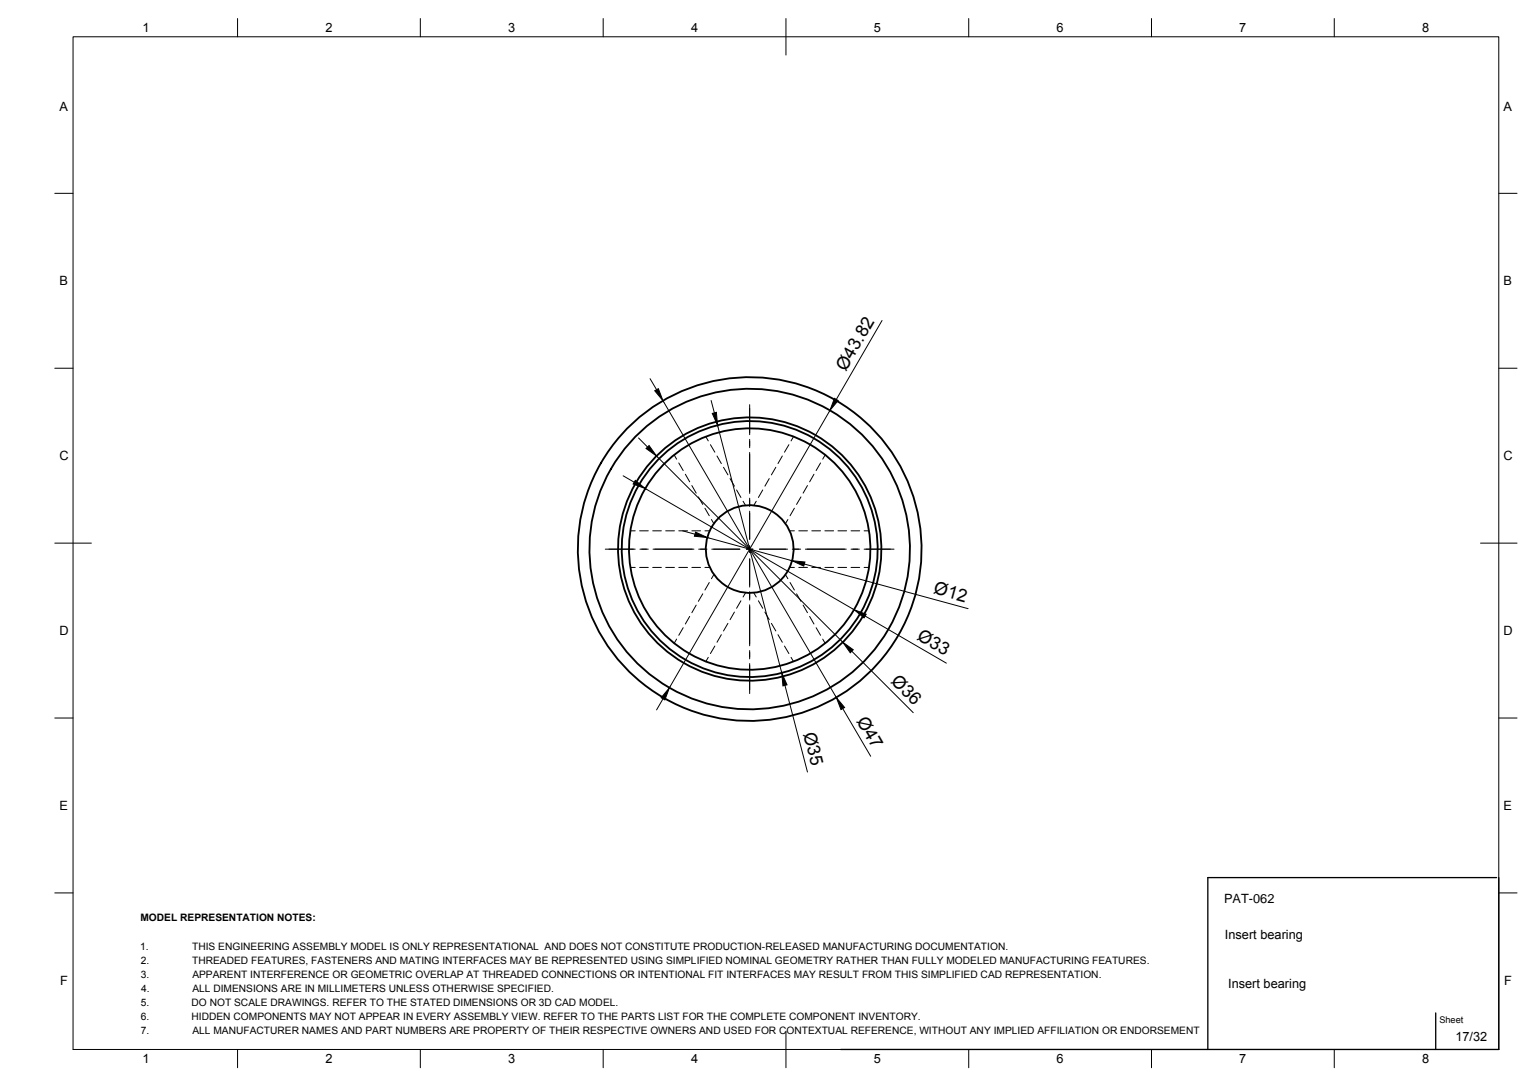
ISO-10303-21;
HEADER;
/* Generated by software containing ST-Developer
 * from STEP Tools, Inc. (www.steptools.com) 
 */

FILE_DESCRIPTION(
/* description */ ('Jaw-coupled motor to shaft test stand'),
/* implementation_level */ '2;1');

FILE_NAME(
/* name */ 'Insert bearing.step',
/* time_stamp */ '2026-10-27T10:46:06-07:00',
/* author */ (''),
/* organization */ (''),
/* preprocessor_version */ 'ST-DEVELOPER v20.2',
/* originating_system */ 'Autodesk Translation Framework v15.17.0.0',
/* authorisation */ '');

FILE_SCHEMA (('AUTOMOTIVE_DESIGN { 1 0 10303 214 3 1 1 }'));
ENDSEC;

DATA;
#10=MECHANICAL_DESIGN_GEOMETRIC_PRESENTATION_REPRESENTATION('',(#354,#355),#19361);
#227=B_SPLINE_CURVE_WITH_KNOTS('',3,(#16151,#16152,#16153,#16154,#16155,
#16156,#16157,#16158,#16159,#16160),.UNSPECIFIED.,.F.,.F.,(4,2,2,2,4),(1.13193471301885,
1.22626174930539,1.32058878559194,1.41491753480854,1.50924628402513),
 .UNSPECIFIED.);
#228=B_SPLINE_CURVE_WITH_KNOTS('',3,(#16162,#16163,#16164,#16165,#16166,
#16167,#16168,#16169,#16170,#16171,#16172,#16173,#16174,#16175,#16176,#16177,
#16178,#16179),.UNSPECIFIED.,.F.,.F.,(4,2,2,2,2,2,2,2,4),(0.377311571006283,
0.471638607292829,0.565965643579376,0.66029439279597,0.754623142012565,
0.84895189122916,0.943280640445754,1.0376076767323,1.13193471301885),
 .UNSPECIFIED.);
#229=B_SPLINE_CURVE_WITH_KNOTS('',3,(#16180,#16181,#16182,#16183,#16184,
#16185,#16186,#16187,#16188,#16189),.UNSPECIFIED.,.F.,.F.,(4,2,2,2,4),(1.50924628402513,
1.60357503324173,1.69790378245832,1.79223081874487,1.88655785503141),
 .UNSPECIFIED.);
#230=B_SPLINE_CURVE_WITH_KNOTS('',3,(#16192,#16193,#16194,#16195,#16196,
#16197,#16198,#16199,#16200,#16201,#16202,#16203,#16204,#16205,#16206,#16207,
#16208,#16209,#16210,#16211,#16212,#16213,#16214,#16215,#16216,#16217,#16218,
#16219,#16220,#16221,#16222,#16223,#16224,#16225),.UNSPECIFIED.,.T.,.F.,
(4,2,2,2,2,2,2,2,2,2,2,2,2,2,2,2,4),(0.,0.0955080856649705,0.191016171329941,
0.286408845249646,0.38180151916935,0.477194193089055,0.572586867008759,
0.66809495267373,0.763603038338701,0.859111124003671,0.954619209668642,
1.05001188358835,1.14540455750805,1.24079723142776,1.33618990534746,1.43169799101243,
1.5272060766774),.UNSPECIFIED.);
#231=B_SPLINE_CURVE_WITH_KNOTS('',3,(#16228,#16229,#16230,#16231,#16232,
#16233,#16234,#16235,#16236,#16237,#16238,#16239,#16240,#16241,#16242,#16243,
#16244,#16245,#16246,#16247,#16248,#16249,#16250,#16251,#16252,#16253,#16254,
#16255,#16256,#16257,#16258,#16259,#16260,#16261),.UNSPECIFIED.,.T.,.F.,
(4,2,2,2,2,2,2,2,2,2,2,2,2,2,2,2,4),(0.,0.0955080856649706,0.191016171329941,
0.286408845249646,0.381801519169351,0.477194193089055,0.57258686700876,
0.668094952673731,0.763603038338701,0.859111124003672,0.954619209668642,
1.05001188358835,1.14540455750805,1.24079723142776,1.33618990534746,1.43169799101243,
1.5272060766774),.UNSPECIFIED.);
#232=B_SPLINE_CURVE_WITH_KNOTS('',3,(#16265,#16266,#16267,#16268,#16269,
#16270,#16271,#16272,#16273,#16274),.UNSPECIFIED.,.F.,.F.,(4,2,2,2,4),(1.13193471301885,
1.22626174930539,1.32058878559194,1.41491753480854,1.50924628402513),
 .UNSPECIFIED.);
#233=B_SPLINE_CURVE_WITH_KNOTS('',3,(#16276,#16277,#16278,#16279,#16280,
#16281,#16282,#16283,#16284,#16285,#16286,#16287,#16288,#16289,#16290,#16291,
#16292,#16293),.UNSPECIFIED.,.F.,.F.,(4,2,2,2,2,2,2,2,4),(0.377311571006283,
0.47163860729283,0.565965643579376,0.660294392795971,0.754623142012565,
0.84895189122916,0.943280640445755,1.0376076767323,1.13193471301885),
 .UNSPECIFIED.);
#234=B_SPLINE_CURVE_WITH_KNOTS('',3,(#16294,#16295,#16296,#16297,#16298,
#16299,#16300,#16301,#16302,#16303),.UNSPECIFIED.,.F.,.F.,(4,2,2,2,4),(1.50924628402513,
1.60357503324173,1.69790378245832,1.79223081874487,1.88655785503141),
 .UNSPECIFIED.);
#235=B_SPLINE_CURVE_WITH_KNOTS('',3,(#16312,#16313,#16314,#16315,#16316,
#16317,#16318,#16319,#16320,#16321,#16322,#16323,#16324,#16325,#16326,#16327,
#16328,#16329),.UNSPECIFIED.,.F.,.F.,(4,2,2,2,2,2,2,2,4),(0.377311571006282,
0.471638607292829,0.565965643579376,0.660294392795971,0.754623142012565,
0.84895189122916,0.943280640445754,1.0376076767323,1.13193471301885),
 .UNSPECIFIED.);
#236=B_SPLINE_CURVE_WITH_KNOTS('',3,(#16331,#16332,#16333,#16334,#16335,
#16336,#16337,#16338,#16339,#16340),.UNSPECIFIED.,.F.,.F.,(4,2,2,2,4),(1.13193471301885,
1.22626174930539,1.32058878559194,1.41491753480854,1.50924628402513),
 .UNSPECIFIED.);
#237=B_SPLINE_CURVE_WITH_KNOTS('',3,(#16341,#16342,#16343,#16344,#16345,
#16346,#16347,#16348,#16349,#16350),.UNSPECIFIED.,.F.,.F.,(4,2,2,2,4),(1.50924628402513,
1.60357503324172,1.69790378245832,1.79223081874487,1.88655785503141),
 .UNSPECIFIED.);
#238=B_SPLINE_CURVE_WITH_KNOTS('',3,(#16353,#16354,#16355,#16356,#16357,
#16358,#16359,#16360,#16361,#16362,#16363,#16364,#16365,#16366,#16367,#16368,
#16369,#16370),.UNSPECIFIED.,.F.,.F.,(4,2,2,2,2,2,2,2,4),(0.377311571006283,
0.47163860729283,0.565965643579376,0.660294392795971,0.754623142012565,
0.84895189122916,0.943280640445754,1.0376076767323,1.13193471301885),
 .UNSPECIFIED.);
#239=B_SPLINE_CURVE_WITH_KNOTS('',3,(#16372,#16373,#16374,#16375,#16376,
#16377,#16378,#16379,#16380,#16381),.UNSPECIFIED.,.F.,.F.,(4,2,2,2,4),(1.13193471301885,
1.22626174930539,1.32058878559194,1.41491753480854,1.50924628402513),
 .UNSPECIFIED.);
#240=B_SPLINE_CURVE_WITH_KNOTS('',3,(#16382,#16383,#16384,#16385,#16386,
#16387,#16388,#16389,#16390,#16391),.UNSPECIFIED.,.F.,.F.,(4,2,2,2,4),(1.50924628402513,
1.60357503324173,1.69790378245832,1.79223081874487,1.88655785503141),
 .UNSPECIFIED.);
#241=B_SPLINE_CURVE_WITH_KNOTS('',3,(#16394,#16395,#16396,#16397,#16398,
#16399,#16400,#16401,#16402,#16403,#16404,#16405,#16406,#16407,#16408,#16409,
#16410,#16411),.UNSPECIFIED.,.F.,.F.,(4,2,2,2,2,2,2,2,4),(0.377311571006282,
0.471638607292829,0.565965643579376,0.66029439279597,0.754623142012565,
0.84895189122916,0.943280640445754,1.0376076767323,1.13193471301885),
 .UNSPECIFIED.);
#242=B_SPLINE_CURVE_WITH_KNOTS('',3,(#16413,#16414,#16415,#16416,#16417,
#16418,#16419,#16420,#16421,#16422),.UNSPECIFIED.,.F.,.F.,(4,2,2,2,4),(1.13193471301885,
1.22626174930539,1.32058878559194,1.41491753480854,1.50924628402513),
 .UNSPECIFIED.);
#243=B_SPLINE_CURVE_WITH_KNOTS('',3,(#16423,#16424,#16425,#16426,#16427,
#16428,#16429,#16430,#16431,#16432),.UNSPECIFIED.,.F.,.F.,(4,2,2,2,4),(1.50924628402513,
1.60357503324172,1.69790378245832,1.79223081874487,1.88655785503141),
 .UNSPECIFIED.);
#244=B_SPLINE_CURVE_WITH_KNOTS('',3,(#16435,#16436,#16437,#16438,#16439,
#16440,#16441,#16442,#16443,#16444,#16445,#16446,#16447,#16448,#16449,#16450,
#16451,#16452),.UNSPECIFIED.,.F.,.F.,(4,2,2,2,2,2,2,2,4),(0.377311571006283,
0.471638607292829,0.565965643579376,0.660294392795971,0.754623142012565,
0.84895189122916,0.943280640445755,1.0376076767323,1.13193471301885),
 .UNSPECIFIED.);
#245=B_SPLINE_CURVE_WITH_KNOTS('',3,(#16454,#16455,#16456,#16457,#16458,
#16459,#16460,#16461,#16462,#16463),.UNSPECIFIED.,.F.,.F.,(4,2,2,2,4),(1.13193471301885,
1.22626174930539,1.32058878559194,1.41491753480854,1.50924628402513),
 .UNSPECIFIED.);
#246=B_SPLINE_CURVE_WITH_KNOTS('',3,(#16464,#16465,#16466,#16467,#16468,
#16469,#16470,#16471,#16472,#16473),.UNSPECIFIED.,.F.,.F.,(4,2,2,2,4),(1.50924628402513,
1.60357503324172,1.69790378245832,1.79223081874487,1.88655785503141),
 .UNSPECIFIED.);
#247=B_SPLINE_CURVE_WITH_KNOTS('',3,(#16477,#16478,#16479,#16480,#16481,
#16482,#16483,#16484,#16485,#16486,#16487,#16488,#16489,#16490,#16491,#16492,
#16493,#16494,#16495,#16496,#16497,#16498,#16499,#16500,#16501,#16502,#16503,
#16504,#16505,#16506,#16507,#16508,#16509,#16510),.UNSPECIFIED.,.T.,.F.,
(4,2,2,2,2,2,2,2,2,2,2,2,2,2,2,2,4),(0.,0.0955080856649705,0.191016171329941,
0.286408845249646,0.38180151916935,0.477194193089055,0.572586867008759,
0.66809495267373,0.7636030383387,0.859111124003671,0.954619209668642,1.05001188358835,
1.14540455750805,1.24079723142776,1.33618990534746,1.43169799101243,1.5272060766774),
 .UNSPECIFIED.);
#248=B_SPLINE_CURVE_WITH_KNOTS('',3,(#16513,#16514,#16515,#16516,#16517,
#16518,#16519,#16520,#16521,#16522,#16523,#16524,#16525,#16526,#16527,#16528,
#16529,#16530,#16531,#16532,#16533,#16534,#16535,#16536,#16537,#16538,#16539,
#16540,#16541,#16542,#16543,#16544,#16545,#16546),.UNSPECIFIED.,.T.,.F.,
(4,2,2,2,2,2,2,2,2,2,2,2,2,2,2,2,4),(0.,0.0955080856649706,0.191016171329941,
0.286408845249646,0.381801519169351,0.477194193089055,0.57258686700876,
0.668094952673731,0.763603038338701,0.859111124003672,0.954619209668642,
1.05001188358835,1.14540455750805,1.24079723142776,1.33618990534746,1.43169799101243,
1.5272060766774),.UNSPECIFIED.);
#249=B_SPLINE_CURVE_WITH_KNOTS('',3,(#16551,#16552,#16553,#16554,#16555,
#16556,#16557,#16558,#16559,#16560,#16561,#16562,#16563,#16564,#16565,#16566,
#16567,#16568,#16569,#16570,#16571,#16572,#16573,#16574,#16575,#16576,#16577,
#16578,#16579,#16580,#16581,#16582,#16583,#16584),.UNSPECIFIED.,.T.,.F.,
(4,2,2,2,2,2,2,2,2,2,2,2,2,2,2,2,4),(0.,0.0955080856649705,0.191016171329941,
0.286408845249646,0.38180151916935,0.477194193089055,0.572586867008759,
0.66809495267373,0.7636030383387,0.859111124003671,0.954619209668642,1.05001188358835,
1.14540455750805,1.24079723142776,1.33618990534746,1.43169799101243,1.5272060766774),
 .UNSPECIFIED.);
#250=B_SPLINE_CURVE_WITH_KNOTS('',3,(#16587,#16588,#16589,#16590,#16591,
#16592,#16593,#16594,#16595,#16596,#16597,#16598,#16599,#16600,#16601,#16602,
#16603,#16604,#16605,#16606,#16607,#16608,#16609,#16610,#16611,#16612,#16613,
#16614,#16615,#16616,#16617,#16618,#16619,#16620),.UNSPECIFIED.,.T.,.F.,
(4,2,2,2,2,2,2,2,2,2,2,2,2,2,2,2,4),(0.,0.0955080856649706,0.191016171329941,
0.286408845249646,0.381801519169351,0.477194193089055,0.57258686700876,
0.668094952673731,0.763603038338701,0.859111124003672,0.954619209668642,
1.05001188358835,1.14540455750805,1.24079723142776,1.33618990534746,1.43169799101243,
1.5272060766774),.UNSPECIFIED.);
#275=SPHERICAL_SURFACE('',#11636,2.35);
#290=SHAPE_REPRESENTATION_RELATIONSHIP('SRR','None',#19505,#322);
#322=ADVANCED_BREP_SHAPE_REPRESENTATION('',(#387,#388),#19341);
#354=STYLED_ITEM('',(#19746),#387);
#355=STYLED_ITEM('',(#19746),#388);
#387=MANIFOLD_SOLID_BREP('Body1',#10998);
#388=MANIFOLD_SOLID_BREP('Body2',#10999);
#460=FACE_BOUND('',#1850,.T.);
#461=FACE_BOUND('',#1852,.T.);
#462=FACE_BOUND('',#1853,.T.);
#463=FACE_BOUND('',#1855,.T.);
#464=FACE_BOUND('',#1859,.T.);
#465=FACE_BOUND('',#1860,.T.);
#466=FACE_BOUND('',#1861,.T.);
#467=FACE_BOUND('',#1862,.T.);
#468=FACE_BOUND('',#1863,.T.);
#469=FACE_BOUND('',#1864,.T.);
#470=FACE_BOUND('',#1870,.T.);
#471=FACE_BOUND('',#1872,.T.);
#472=FACE_BOUND('',#1875,.T.);
#473=FACE_BOUND('',#1877,.T.);
#474=FACE_BOUND('',#1878,.T.);
#475=FACE_BOUND('',#1879,.T.);
#476=FACE_BOUND('',#1880,.T.);
#477=FACE_BOUND('',#1881,.T.);
#478=FACE_BOUND('',#1882,.T.);
#623=PLANE('',#11634);
#624=PLANE('',#11639);
#625=PLANE('',#11649);
#626=PLANE('',#11651);
#627=PLANE('',#11655);
#1171=FACE_OUTER_BOUND('',#1848,.T.);
#1172=FACE_OUTER_BOUND('',#1849,.T.);
#1173=FACE_OUTER_BOUND('',#1851,.T.);
#1174=FACE_OUTER_BOUND('',#1854,.T.);
#1175=FACE_OUTER_BOUND('',#1856,.T.);
#1176=FACE_OUTER_BOUND('',#1857,.T.);
#1177=FACE_OUTER_BOUND('',#1858,.T.);
#1178=FACE_OUTER_BOUND('',#1865,.T.);
#1179=FACE_OUTER_BOUND('',#1866,.T.);
#1180=FACE_OUTER_BOUND('',#1867,.T.);
#1181=FACE_OUTER_BOUND('',#1868,.T.);
#1182=FACE_OUTER_BOUND('',#1869,.T.);
#1183=FACE_OUTER_BOUND('',#1871,.T.);
#1184=FACE_OUTER_BOUND('',#1873,.T.);
#1185=FACE_OUTER_BOUND('',#1874,.T.);
#1186=FACE_OUTER_BOUND('',#1876,.T.);
#1848=EDGE_LOOP('',(#7990,#7991,#7992,#7993));
#1849=EDGE_LOOP('',(#7994));
#1850=EDGE_LOOP('',(#7995));
#1851=EDGE_LOOP('',(#7996,#7997));
#1852=EDGE_LOOP('',(#7998));
#1853=EDGE_LOOP('',(#7999));
#1854=EDGE_LOOP('',(#8000));
#1855=EDGE_LOOP('',(#8001));
#1856=EDGE_LOOP('',(#8002,#8003,#8004,#8005,#8006,#8007));
#1857=EDGE_LOOP('',(#8008,#8009,#8010,#8011,#8012,#8013));
#1858=EDGE_LOOP('',(#8014,#8015,#8016,#8017));
#1859=EDGE_LOOP('',(#8018,#8019,#8020));
#1860=EDGE_LOOP('',(#8021,#8022,#8023));
#1861=EDGE_LOOP('',(#8024,#8025,#8026));
#1862=EDGE_LOOP('',(#8027,#8028,#8029));
#1863=EDGE_LOOP('',(#8030,#8031,#8032));
#1864=EDGE_LOOP('',(#8033,#8034,#8035));
#1865=EDGE_LOOP('',(#8036,#8037,#8038,#8039,#8040,#8041));
#1866=EDGE_LOOP('',(#8042,#8043,#8044,#8045,#8046,#8047));
#1867=EDGE_LOOP('',(#8048,#8049,#8050,#8051,#8052,#8053));
#1868=EDGE_LOOP('',(#8054,#8055,#8056,#8057,#8058,#8059));
#1869=EDGE_LOOP('',(#8060));
#1870=EDGE_LOOP('',(#8061));
#1871=EDGE_LOOP('',(#8062));
#1872=EDGE_LOOP('',(#8063));
#1873=EDGE_LOOP('',(#8064,#8065,#8066,#8067));
#1874=EDGE_LOOP('',(#8068));
#1875=EDGE_LOOP('',(#8069));
#1876=EDGE_LOOP('',(#8070,#8071,#8072,#8073));
#1877=EDGE_LOOP('',(#8074));
#1878=EDGE_LOOP('',(#8075));
#1879=EDGE_LOOP('',(#8076));
#1880=EDGE_LOOP('',(#8077));
#1881=EDGE_LOOP('',(#8078));
#1882=EDGE_LOOP('',(#8079));
#2606=LINE('',#16136,#3759);
#2607=LINE('',#16191,#3760);
#2608=LINE('',#16263,#3761);
#2609=LINE('',#16308,#3762);
#2610=LINE('',#16476,#3763);
#2611=LINE('',#16547,#3764);
#2612=LINE('',#16550,#3765);
#2613=LINE('',#16621,#3766);
#2614=LINE('',#16631,#3767);
#2615=LINE('',#16636,#3768);
#3759=VECTOR('',#13091,1.8);
#3760=VECTOR('',#13108,0.25);
#3761=VECTOR('',#13111,0.25);
#3762=VECTOR('',#13116,1.65);
#3763=VECTOR('',#13121,0.25);
#3764=VECTOR('',#13124,0.25);
#3765=VECTOR('',#13127,0.25);
#3766=VECTOR('',#13130,0.25);
#3767=VECTOR('',#13143,1.75);
#3768=VECTOR('',#13150,0.6);
#4772=CIRCLE('',#11632,1.8);
#4773=CIRCLE('',#11633,1.8);
#4774=CIRCLE('',#11635,2.19089023002066);
#4775=CIRCLE('',#11637,2.35);
#4776=CIRCLE('',#11638,2.19089023002066);
#4777=CIRCLE('',#11643,1.65);
#4778=CIRCLE('',#11644,1.65);
#4779=CIRCLE('',#11650,0.6);
#4780=CIRCLE('',#11652,1.75);
#4781=CIRCLE('',#11654,1.75);
#4782=CIRCLE('',#11656,0.6);
#5159=VERTEX_POINT('',#16133);
#5160=VERTEX_POINT('',#16135);
#5161=VERTEX_POINT('',#16139);
#5162=VERTEX_POINT('',#16142);
#5163=VERTEX_POINT('',#16143);
#5164=VERTEX_POINT('',#16145);
#5165=VERTEX_POINT('',#16149);
#5166=VERTEX_POINT('',#16150);
#5167=VERTEX_POINT('',#16161);
#5168=VERTEX_POINT('',#16190);
#5169=VERTEX_POINT('',#16227);
#5170=VERTEX_POINT('',#16262);
#5171=VERTEX_POINT('',#16264);
#5172=VERTEX_POINT('',#16275);
#5173=VERTEX_POINT('',#16305);
#5174=VERTEX_POINT('',#16307);
#5175=VERTEX_POINT('',#16310);
#5176=VERTEX_POINT('',#16311);
#5177=VERTEX_POINT('',#16330);
#5178=VERTEX_POINT('',#16351);
#5179=VERTEX_POINT('',#16352);
#5180=VERTEX_POINT('',#16371);
#5181=VERTEX_POINT('',#16392);
#5182=VERTEX_POINT('',#16393);
#5183=VERTEX_POINT('',#16412);
#5184=VERTEX_POINT('',#16433);
#5185=VERTEX_POINT('',#16434);
#5186=VERTEX_POINT('',#16453);
#5187=VERTEX_POINT('',#16475);
#5188=VERTEX_POINT('',#16512);
#5189=VERTEX_POINT('',#16549);
#5190=VERTEX_POINT('',#16586);
#5191=VERTEX_POINT('',#16623);
#5192=VERTEX_POINT('',#16626);
#5193=VERTEX_POINT('',#16629);
#5194=VERTEX_POINT('',#16633);
#6206=EDGE_CURVE('',#5159,#5159,#4772,.T.);
#6207=EDGE_CURVE('',#5159,#5160,#2606,.T.);
#6208=EDGE_CURVE('',#5160,#5160,#4773,.T.);
#6209=EDGE_CURVE('',#5161,#5161,#4774,.T.);
#6210=EDGE_CURVE('',#5162,#5163,#4775,.T.);
#6211=EDGE_CURVE('',#5164,#5164,#4776,.T.);
#6212=EDGE_CURVE('',#5165,#5166,#227,.T.);
#6213=EDGE_CURVE('',#5167,#5165,#228,.T.);
#6214=EDGE_CURVE('',#5166,#5167,#229,.T.);
#6215=EDGE_CURVE('',#5166,#5168,#2607,.T.);
#6216=EDGE_CURVE('',#5168,#5168,#230,.T.);
#6217=EDGE_CURVE('',#5169,#5169,#231,.T.);
#6218=EDGE_CURVE('',#5169,#5170,#2608,.T.);
#6219=EDGE_CURVE('',#5171,#5170,#232,.T.);
#6220=EDGE_CURVE('',#5172,#5171,#233,.T.);
#6221=EDGE_CURVE('',#5170,#5172,#234,.T.);
#6222=EDGE_CURVE('',#5173,#5173,#4777,.T.);
#6223=EDGE_CURVE('',#5173,#5174,#2609,.T.);
#6224=EDGE_CURVE('',#5174,#5174,#4778,.T.);
#6225=EDGE_CURVE('',#5175,#5176,#235,.T.);
#6226=EDGE_CURVE('',#5176,#5177,#236,.T.);
#6227=EDGE_CURVE('',#5177,#5175,#237,.T.);
#6228=EDGE_CURVE('',#5178,#5179,#238,.T.);
#6229=EDGE_CURVE('',#5179,#5180,#239,.T.);
#6230=EDGE_CURVE('',#5180,#5178,#240,.T.);
#6231=EDGE_CURVE('',#5181,#5182,#241,.T.);
#6232=EDGE_CURVE('',#5182,#5183,#242,.T.);
#6233=EDGE_CURVE('',#5183,#5181,#243,.T.);
#6234=EDGE_CURVE('',#5184,#5185,#244,.T.);
#6235=EDGE_CURVE('',#5185,#5186,#245,.T.);
#6236=EDGE_CURVE('',#5186,#5184,#246,.T.);
#6237=EDGE_CURVE('',#5177,#5187,#2610,.T.);
#6238=EDGE_CURVE('',#5187,#5187,#247,.T.);
#6239=EDGE_CURVE('',#5188,#5188,#248,.T.);
#6240=EDGE_CURVE('',#5188,#5180,#2611,.T.);
#6241=EDGE_CURVE('',#5183,#5189,#2612,.T.);
#6242=EDGE_CURVE('',#5189,#5189,#249,.T.);
#6243=EDGE_CURVE('',#5190,#5190,#250,.T.);
#6244=EDGE_CURVE('',#5190,#5186,#2613,.T.);
#6245=EDGE_CURVE('',#5191,#5191,#4779,.T.);
#6246=EDGE_CURVE('',#5192,#5192,#4780,.T.);
#6247=EDGE_CURVE('',#5193,#5193,#4781,.T.);
#6248=EDGE_CURVE('',#5193,#5192,#2614,.T.);
#6249=EDGE_CURVE('',#5194,#5194,#4782,.T.);
#6250=EDGE_CURVE('',#5194,#5191,#2615,.T.);
#7990=ORIENTED_EDGE('',*,*,#6206,.T.);
#7991=ORIENTED_EDGE('',*,*,#6207,.T.);
#7992=ORIENTED_EDGE('',*,*,#6208,.F.);
#7993=ORIENTED_EDGE('',*,*,#6207,.F.);
#7994=ORIENTED_EDGE('',*,*,#6209,.F.);
#7995=ORIENTED_EDGE('',*,*,#6208,.T.);
#7996=ORIENTED_EDGE('',*,*,#6210,.T.);
#7997=ORIENTED_EDGE('',*,*,#6210,.F.);
#7998=ORIENTED_EDGE('',*,*,#6209,.T.);
#7999=ORIENTED_EDGE('',*,*,#6211,.F.);
#8000=ORIENTED_EDGE('',*,*,#6211,.T.);
#8001=ORIENTED_EDGE('',*,*,#6206,.F.);
#8002=ORIENTED_EDGE('',*,*,#6212,.F.);
#8003=ORIENTED_EDGE('',*,*,#6213,.F.);
#8004=ORIENTED_EDGE('',*,*,#6214,.F.);
#8005=ORIENTED_EDGE('',*,*,#6215,.T.);
#8006=ORIENTED_EDGE('',*,*,#6216,.F.);
#8007=ORIENTED_EDGE('',*,*,#6215,.F.);
#8008=ORIENTED_EDGE('',*,*,#6217,.F.);
#8009=ORIENTED_EDGE('',*,*,#6218,.T.);
#8010=ORIENTED_EDGE('',*,*,#6219,.F.);
#8011=ORIENTED_EDGE('',*,*,#6220,.F.);
#8012=ORIENTED_EDGE('',*,*,#6221,.F.);
#8013=ORIENTED_EDGE('',*,*,#6218,.F.);
#8014=ORIENTED_EDGE('',*,*,#6222,.F.);
#8015=ORIENTED_EDGE('',*,*,#6223,.T.);
#8016=ORIENTED_EDGE('',*,*,#6224,.T.);
#8017=ORIENTED_EDGE('',*,*,#6223,.F.);
#8018=ORIENTED_EDGE('',*,*,#6213,.T.);
#8019=ORIENTED_EDGE('',*,*,#6212,.T.);
#8020=ORIENTED_EDGE('',*,*,#6214,.T.);
#8021=ORIENTED_EDGE('',*,*,#6220,.T.);
#8022=ORIENTED_EDGE('',*,*,#6219,.T.);
#8023=ORIENTED_EDGE('',*,*,#6221,.T.);
#8024=ORIENTED_EDGE('',*,*,#6225,.T.);
#8025=ORIENTED_EDGE('',*,*,#6226,.T.);
#8026=ORIENTED_EDGE('',*,*,#6227,.T.);
#8027=ORIENTED_EDGE('',*,*,#6228,.T.);
#8028=ORIENTED_EDGE('',*,*,#6229,.T.);
#8029=ORIENTED_EDGE('',*,*,#6230,.T.);
#8030=ORIENTED_EDGE('',*,*,#6231,.T.);
#8031=ORIENTED_EDGE('',*,*,#6232,.T.);
#8032=ORIENTED_EDGE('',*,*,#6233,.T.);
#8033=ORIENTED_EDGE('',*,*,#6234,.T.);
#8034=ORIENTED_EDGE('',*,*,#6235,.T.);
#8035=ORIENTED_EDGE('',*,*,#6236,.T.);
#8036=ORIENTED_EDGE('',*,*,#6226,.F.);
#8037=ORIENTED_EDGE('',*,*,#6225,.F.);
#8038=ORIENTED_EDGE('',*,*,#6227,.F.);
#8039=ORIENTED_EDGE('',*,*,#6237,.T.);
#8040=ORIENTED_EDGE('',*,*,#6238,.F.);
#8041=ORIENTED_EDGE('',*,*,#6237,.F.);
#8042=ORIENTED_EDGE('',*,*,#6239,.F.);
#8043=ORIENTED_EDGE('',*,*,#6240,.T.);
#8044=ORIENTED_EDGE('',*,*,#6229,.F.);
#8045=ORIENTED_EDGE('',*,*,#6228,.F.);
#8046=ORIENTED_EDGE('',*,*,#6230,.F.);
#8047=ORIENTED_EDGE('',*,*,#6240,.F.);
#8048=ORIENTED_EDGE('',*,*,#6232,.F.);
#8049=ORIENTED_EDGE('',*,*,#6231,.F.);
#8050=ORIENTED_EDGE('',*,*,#6233,.F.);
#8051=ORIENTED_EDGE('',*,*,#6241,.T.);
#8052=ORIENTED_EDGE('',*,*,#6242,.F.);
#8053=ORIENTED_EDGE('',*,*,#6241,.F.);
#8054=ORIENTED_EDGE('',*,*,#6243,.F.);
#8055=ORIENTED_EDGE('',*,*,#6244,.T.);
#8056=ORIENTED_EDGE('',*,*,#6235,.F.);
#8057=ORIENTED_EDGE('',*,*,#6234,.F.);
#8058=ORIENTED_EDGE('',*,*,#6236,.F.);
#8059=ORIENTED_EDGE('',*,*,#6244,.F.);
#8060=ORIENTED_EDGE('',*,*,#6224,.F.);
#8061=ORIENTED_EDGE('',*,*,#6245,.T.);
#8062=ORIENTED_EDGE('',*,*,#6246,.F.);
#8063=ORIENTED_EDGE('',*,*,#6222,.T.);
#8064=ORIENTED_EDGE('',*,*,#6247,.F.);
#8065=ORIENTED_EDGE('',*,*,#6248,.T.);
#8066=ORIENTED_EDGE('',*,*,#6246,.T.);
#8067=ORIENTED_EDGE('',*,*,#6248,.F.);
#8068=ORIENTED_EDGE('',*,*,#6247,.T.);
#8069=ORIENTED_EDGE('',*,*,#6249,.F.);
#8070=ORIENTED_EDGE('',*,*,#6249,.T.);
#8071=ORIENTED_EDGE('',*,*,#6250,.T.);
#8072=ORIENTED_EDGE('',*,*,#6245,.F.);
#8073=ORIENTED_EDGE('',*,*,#6250,.F.);
#8074=ORIENTED_EDGE('',*,*,#6217,.T.);
#8075=ORIENTED_EDGE('',*,*,#6216,.T.);
#8076=ORIENTED_EDGE('',*,*,#6239,.T.);
#8077=ORIENTED_EDGE('',*,*,#6238,.T.);
#8078=ORIENTED_EDGE('',*,*,#6243,.T.);
#8079=ORIENTED_EDGE('',*,*,#6242,.T.);
#10311=CYLINDRICAL_SURFACE('',#11631,1.8);
#10312=CYLINDRICAL_SURFACE('',#11640,0.25);
#10313=CYLINDRICAL_SURFACE('',#11641,0.25);
#10314=CYLINDRICAL_SURFACE('',#11642,1.65);
#10315=CYLINDRICAL_SURFACE('',#11645,0.25);
#10316=CYLINDRICAL_SURFACE('',#11646,0.25);
#10317=CYLINDRICAL_SURFACE('',#11647,0.25);
#10318=CYLINDRICAL_SURFACE('',#11648,0.25);
#10319=CYLINDRICAL_SURFACE('',#11653,1.75);
#10320=CYLINDRICAL_SURFACE('',#11657,0.6);
#10513=ADVANCED_FACE('',(#1171),#10311,.F.);
#10514=ADVANCED_FACE('',(#1172,#460),#623,.T.);
#10515=ADVANCED_FACE('',(#1173,#461,#462),#275,.T.);
#10516=ADVANCED_FACE('',(#1174,#463),#624,.T.);
#10517=ADVANCED_FACE('',(#1175),#10312,.F.);
#10518=ADVANCED_FACE('',(#1176),#10313,.F.);
#10519=ADVANCED_FACE('',(#1177,#464,#465,#466,#467,#468,#469),#10314,.T.);
#10520=ADVANCED_FACE('',(#1178),#10315,.F.);
#10521=ADVANCED_FACE('',(#1179),#10316,.F.);
#10522=ADVANCED_FACE('',(#1180),#10317,.F.);
#10523=ADVANCED_FACE('',(#1181),#10318,.F.);
#10524=ADVANCED_FACE('',(#1182,#470),#625,.T.);
#10525=ADVANCED_FACE('',(#1183,#471),#626,.T.);
#10526=ADVANCED_FACE('',(#1184),#10319,.T.);
#10527=ADVANCED_FACE('',(#1185,#472),#627,.T.);
#10528=ADVANCED_FACE('',(#1186,#473,#474,#475,#476,#477,#478),#10320,.F.);
#10998=CLOSED_SHELL('',(#10513,#10514,#10515,#10516));
#10999=CLOSED_SHELL('',(#10517,#10518,#10519,#10520,#10521,#10522,#10523,
#10524,#10525,#10526,#10527,#10528));
#11630=AXIS2_PLACEMENT_3D('',#16131,#13085,#13086);
#11631=AXIS2_PLACEMENT_3D('',#16132,#13087,#13088);
#11632=AXIS2_PLACEMENT_3D('',#16134,#13089,#13090);
#11633=AXIS2_PLACEMENT_3D('',#16137,#13092,#13093);
#11634=AXIS2_PLACEMENT_3D('',#16138,#13094,#13095);
#11635=AXIS2_PLACEMENT_3D('',#16140,#13096,#13097);
#11636=AXIS2_PLACEMENT_3D('',#16141,#13098,#13099);
#11637=AXIS2_PLACEMENT_3D('',#16144,#13100,#13101);
#11638=AXIS2_PLACEMENT_3D('',#16146,#13102,#13103);
#11639=AXIS2_PLACEMENT_3D('',#16147,#13104,#13105);
#11640=AXIS2_PLACEMENT_3D('',#16148,#13106,#13107);
#11641=AXIS2_PLACEMENT_3D('',#16226,#13109,#13110);
#11642=AXIS2_PLACEMENT_3D('',#16304,#13112,#13113);
#11643=AXIS2_PLACEMENT_3D('',#16306,#13114,#13115);
#11644=AXIS2_PLACEMENT_3D('',#16309,#13117,#13118);
#11645=AXIS2_PLACEMENT_3D('',#16474,#13119,#13120);
#11646=AXIS2_PLACEMENT_3D('',#16511,#13122,#13123);
#11647=AXIS2_PLACEMENT_3D('',#16548,#13125,#13126);
#11648=AXIS2_PLACEMENT_3D('',#16585,#13128,#13129);
#11649=AXIS2_PLACEMENT_3D('',#16622,#13131,#13132);
#11650=AXIS2_PLACEMENT_3D('',#16624,#13133,#13134);
#11651=AXIS2_PLACEMENT_3D('',#16625,#13135,#13136);
#11652=AXIS2_PLACEMENT_3D('',#16627,#13137,#13138);
#11653=AXIS2_PLACEMENT_3D('',#16628,#13139,#13140);
#11654=AXIS2_PLACEMENT_3D('',#16630,#13141,#13142);
#11655=AXIS2_PLACEMENT_3D('',#16632,#13144,#13145);
#11656=AXIS2_PLACEMENT_3D('',#16634,#13146,#13147);
#11657=AXIS2_PLACEMENT_3D('',#16635,#13148,#13149);
#13085=DIRECTION('axis',(0.,0.,1.));
#13086=DIRECTION('refdir',(1.,0.,0.));
#13087=DIRECTION('center_axis',(0.,-1.,0.));
#13088=DIRECTION('ref_axis',(1.,0.,0.));
#13089=DIRECTION('center_axis',(0.,-1.,0.));
#13090=DIRECTION('ref_axis',(1.,0.,0.));
#13091=DIRECTION('',(0.,1.,0.));
#13092=DIRECTION('center_axis',(0.,-1.,0.));
#13093=DIRECTION('ref_axis',(1.,0.,0.));
#13094=DIRECTION('center_axis',(0.,1.,0.));
#13095=DIRECTION('ref_axis',(0.,0.,1.));
#13096=DIRECTION('center_axis',(0.,-1.,0.));
#13097=DIRECTION('ref_axis',(1.,0.,0.));
#13098=DIRECTION('center_axis',(6.12323399573677E-17,0.,1.));
#13099=DIRECTION('ref_axis',(1.,0.,0.));
#13100=DIRECTION('center_axis',(1.22464679914735E-16,-1.,0.));
#13101=DIRECTION('ref_axis',(-1.,-1.22464679914735E-16,0.));
#13102=DIRECTION('center_axis',(0.,-1.,0.));
#13103=DIRECTION('ref_axis',(1.,0.,0.));
#13104=DIRECTION('center_axis',(0.,-1.,0.));
#13105=DIRECTION('ref_axis',(0.,0.,-1.));
#13106=DIRECTION('center_axis',(-0.866025403784438,0.,-0.5));
#13107=DIRECTION('ref_axis',(-0.5,0.,0.866025403784438));
#13108=DIRECTION('',(-0.866025403784438,0.,-0.5));
#13109=DIRECTION('center_axis',(-0.866025403784438,0.,-0.5));
#13110=DIRECTION('ref_axis',(-0.5,0.,0.866025403784438));
#13111=DIRECTION('',(-0.866025403784438,0.,-0.5));
#13112=DIRECTION('center_axis',(0.,-1.,0.));
#13113=DIRECTION('ref_axis',(1.,0.,0.));
#13114=DIRECTION('center_axis',(0.,-1.,0.));
#13115=DIRECTION('ref_axis',(1.,0.,0.));
#13116=DIRECTION('',(0.,1.,0.));
#13117=DIRECTION('center_axis',(0.,-1.,0.));
#13118=DIRECTION('ref_axis',(1.,0.,0.));
#13119=DIRECTION('center_axis',(0.866025403784439,0.,-0.5));
#13120=DIRECTION('ref_axis',(-0.5,0.,-0.866025403784439));
#13121=DIRECTION('',(0.866025403784439,0.,-0.5));
#13122=DIRECTION('center_axis',(0.866025403784439,0.,-0.5));
#13123=DIRECTION('ref_axis',(-0.5,0.,-0.866025403784439));
#13124=DIRECTION('',(0.866025403784439,0.,-0.5));
#13125=DIRECTION('center_axis',(0.,0.,1.));
#13126=DIRECTION('ref_axis',(1.,0.,0.));
#13127=DIRECTION('',(0.,0.,1.));
#13128=DIRECTION('center_axis',(0.,0.,1.));
#13129=DIRECTION('ref_axis',(1.,0.,0.));
#13130=DIRECTION('',(0.,0.,1.));
#13131=DIRECTION('center_axis',(0.,1.,0.));
#13132=DIRECTION('ref_axis',(0.,0.,1.));
#13133=DIRECTION('center_axis',(0.,-1.,0.));
#13134=DIRECTION('ref_axis',(1.,0.,0.));
#13135=DIRECTION('center_axis',(0.,1.,0.));
#13136=DIRECTION('ref_axis',(0.,0.,1.));
#13137=DIRECTION('center_axis',(0.,-1.,0.));
#13138=DIRECTION('ref_axis',(1.,0.,0.));
#13139=DIRECTION('center_axis',(0.,-1.,0.));
#13140=DIRECTION('ref_axis',(1.,0.,0.));
#13141=DIRECTION('center_axis',(0.,-1.,0.));
#13142=DIRECTION('ref_axis',(1.,0.,0.));
#13143=DIRECTION('',(0.,1.,0.));
#13144=DIRECTION('center_axis',(0.,-1.,0.));
#13145=DIRECTION('ref_axis',(0.,0.,-1.));
#13146=DIRECTION('center_axis',(0.,-1.,0.));
#13147=DIRECTION('ref_axis',(1.,0.,0.));
#13148=DIRECTION('center_axis',(0.,-1.,0.));
#13149=DIRECTION('ref_axis',(1.,0.,0.));
#13150=DIRECTION('',(0.,1.,0.));
#16131=CARTESIAN_POINT('',(0.,0.,0.));
#16132=CARTESIAN_POINT('Origin',(0.,0.,0.));
#16133=CARTESIAN_POINT('',(-1.8,-0.85,-2.20436423846524E-16));
#16134=CARTESIAN_POINT('Origin',(0.,-0.85,0.));
#16135=CARTESIAN_POINT('',(-1.8,0.85,-2.20436423846524E-16));
#16136=CARTESIAN_POINT('',(-1.8,0.,-2.20436423846524E-16));
#16137=CARTESIAN_POINT('Origin',(0.,0.85,0.));
#16138=CARTESIAN_POINT('Origin',(2.19089023002066,0.85,0.));
#16139=CARTESIAN_POINT('',(2.19089023002066,0.85,0.));
#16140=CARTESIAN_POINT('Origin',(0.,0.85,0.));
#16141=CARTESIAN_POINT('Origin',(3.99680288865056E-15,0.,0.));
#16142=CARTESIAN_POINT('',(3.85290688975075E-15,-1.76221774462768E-32,2.35));
#16143=CARTESIAN_POINT('',(3.85290688975075E-15,-1.76221774462768E-32,-2.35));
#16144=CARTESIAN_POINT('Origin',(3.99680288865056E-15,0.,0.));
#16145=CARTESIAN_POINT('',(2.19089023002066,-0.85,0.));
#16146=CARTESIAN_POINT('Origin',(0.,-0.85,0.));
#16147=CARTESIAN_POINT('Origin',(1.8,-0.85,0.));
#16148=CARTESIAN_POINT('Origin',(0.,1.55,0.));
#16149=CARTESIAN_POINT('',(1.42894191624432,1.8,0.825000000000001));
#16150=CARTESIAN_POINT('',(1.53744468918255,1.55,0.598968970568896));
#16151=CARTESIAN_POINT('Ctrl Pts',(1.42894191624432,1.8,0.825000000000001));
#16152=CARTESIAN_POINT('Ctrl Pts',(1.44466308895875,1.8,0.797770130104052));
#16153=CARTESIAN_POINT('Ctrl Pts',(1.46055812562105,1.79370633789704,0.768258557763732));
#16154=CARTESIAN_POINT('Ctrl Pts',(1.48824888379079,1.76817777258318,0.713138492740816));
#16155=CARTESIAN_POINT('Ctrl Pts',(1.50008999307766,1.74894552961493,0.687551581002689));
#16156=CARTESIAN_POINT('Ctrl Pts',(1.51812136280714,1.70460745840382,0.646764802471699));
#16157=CARTESIAN_POINT('Ctrl Pts',(1.52552758004446,1.67652816181843,0.628833667319578));
#16158=CARTESIAN_POINT('Ctrl Pts',(1.53516661651472,1.61494799959182,0.604921184808251));
#16159=CARTESIAN_POINT('Ctrl Pts',(1.53744468918255,1.58144291640553,0.598968970568896));
#16160=CARTESIAN_POINT('Ctrl Pts',(1.53744468918255,1.55,0.598968970568896));
#16161=CARTESIAN_POINT('',(1.42894191624432,1.3,0.825000000000001));
#16162=CARTESIAN_POINT('Ctrl Pts',(1.42894191624432,1.3,0.825000000000001));
#16163=CARTESIAN_POINT('Ctrl Pts',(1.4132207435299,1.3,0.852229869895949));
#16164=CARTESIAN_POINT('Ctrl Pts',(1.39561049050871,1.30629366210296,0.880751161609749));
#16165=CARTESIAN_POINT('Ctrl Pts',(1.36172049302549,1.33182222741682,0.932292094146256));
#16166=CARTESIAN_POINT('Ctrl Pts',(1.34548213209931,1.35105447038507,0.955340251466734));
#16167=CARTESIAN_POINT('Ctrl Pts',(1.31917543061769,1.39539254159618,0.99134926498299));
#16168=CARTESIAN_POINT('Ctrl Pts',(1.30734972067592,1.42347183818157,1.00672880483252));
#16169=CARTESIAN_POINT('Ctrl Pts',(1.29146042158868,1.48505200040818,1.02703269653942));
#16170=CARTESIAN_POINT('Ctrl Pts',(1.28744468918255,1.51855708359447,1.03198167246111));
#16171=CARTESIAN_POINT('Ctrl Pts',(1.28744468918255,1.58144291640553,1.03198167246111));
#16172=CARTESIAN_POINT('Ctrl Pts',(1.29146042158868,1.61494799959182,1.02703269653942));
#16173=CARTESIAN_POINT('Ctrl Pts',(1.30734972067592,1.67652816181843,1.00672880483252));
#16174=CARTESIAN_POINT('Ctrl Pts',(1.31917543061769,1.70460745840382,0.991349264982991));
#16175=CARTESIAN_POINT('Ctrl Pts',(1.34548213209931,1.74894552961493,0.955340251466735));
#16176=CARTESIAN_POINT('Ctrl Pts',(1.36172049302549,1.76817777258318,0.932292094146256));
#16177=CARTESIAN_POINT('Ctrl Pts',(1.39561049050871,1.79370633789704,0.880751161609749));
#16178=CARTESIAN_POINT('Ctrl Pts',(1.4132207435299,1.8,0.85222986989595));
#16179=CARTESIAN_POINT('Ctrl Pts',(1.42894191624432,1.8,0.825000000000001));
#16180=CARTESIAN_POINT('Ctrl Pts',(1.53744468918255,1.55,0.598968970568896));
#16181=CARTESIAN_POINT('Ctrl Pts',(1.53744468918255,1.51855708359447,0.598968970568896));
#16182=CARTESIAN_POINT('Ctrl Pts',(1.53516661651472,1.48505200040818,0.60492118480825));
#16183=CARTESIAN_POINT('Ctrl Pts',(1.52552758004446,1.42347183818157,0.628833667319578));
#16184=CARTESIAN_POINT('Ctrl Pts',(1.51812136280714,1.39539254159618,0.646764802471699));
#16185=CARTESIAN_POINT('Ctrl Pts',(1.50008999307766,1.35105447038507,0.687551581002689));
#16186=CARTESIAN_POINT('Ctrl Pts',(1.48824888379079,1.33182222741682,0.713138492740816));
#16187=CARTESIAN_POINT('Ctrl Pts',(1.46055812562105,1.30629366210296,0.768258557763732));
#16188=CARTESIAN_POINT('Ctrl Pts',(1.44466308895875,1.3,0.797770130104052));
#16189=CARTESIAN_POINT('Ctrl Pts',(1.42894191624432,1.3,0.825000000000001));
#16190=CARTESIAN_POINT('',(0.59736109069228,1.55,0.0562114519197835));
#16191=CARTESIAN_POINT('',(0.125,1.55,-0.21650635094611));
#16192=CARTESIAN_POINT('Ctrl Pts',(0.59736109069228,1.55,0.0562114519197835));
#16193=CARTESIAN_POINT('Ctrl Pts',(0.59736109069228,1.58183602855499,0.0562114519197835));
#16194=CARTESIAN_POINT('Ctrl Pts',(0.596809586309859,1.61548166177648,0.0633319361811907));
#16195=CARTESIAN_POINT('Ctrl Pts',(0.593243052195919,1.67693412158597,0.0908585874761106));
#16196=CARTESIAN_POINT('Ctrl Pts',(0.590063593315144,1.70478184753241,0.111151766652641));
#16197=CARTESIAN_POINT('Ctrl Pts',(0.579820497891285,1.74874496453875,0.15600214762839));
#16198=CARTESIAN_POINT('Ctrl Pts',(0.572042315803119,1.76792916820474,0.183678633836535));
#16199=CARTESIAN_POINT('Ctrl Pts',(0.549947124580676,1.79356669468566,0.241926459727039));
#16200=CARTESIAN_POINT('Ctrl Pts',(0.53551402125728,1.8,0.27246250701687));
#16201=CARTESIAN_POINT('Ctrl Pts',(0.503716463284046,1.8,0.32753749298313));
#16202=CARTESIAN_POINT('Ctrl Pts',(0.484488022261586,1.79356669468566,0.355304950761552));
#16203=CARTESIAN_POINT('Ctrl Pts',(0.445091520936419,1.76792916820474,0.403563860606914));
#16204=CARTESIAN_POINT('Ctrl Pts',(0.425012071836758,1.74874496453875,0.4241382069946));
#16205=CARTESIAN_POINT('Ctrl Pts',(0.391292050254278,1.70478184753241,0.455434178332924));
#16206=CARTESIAN_POINT('Ctrl Pts',(0.375307371004241,1.67693412158597,0.468334260082228));
#16207=CARTESIAN_POINT('Ctrl Pts',(0.353251858758695,1.61548166177647,0.485186294875824));
#16208=CARTESIAN_POINT('Ctrl Pts',(0.347361090692279,1.58183602855499,0.489224153812003));
#16209=CARTESIAN_POINT('Ctrl Pts',(0.347361090692279,1.51816397144501,0.489224153812003));
#16210=CARTESIAN_POINT('Ctrl Pts',(0.353251858758695,1.48451833822352,0.485186294875824));
#16211=CARTESIAN_POINT('Ctrl Pts',(0.375307371004241,1.42306587841403,0.468334260082228));
#16212=CARTESIAN_POINT('Ctrl Pts',(0.391292050254278,1.39521815246759,0.455434178332924));
#16213=CARTESIAN_POINT('Ctrl Pts',(0.425012071836758,1.35125503546125,0.4241382069946));
#16214=CARTESIAN_POINT('Ctrl Pts',(0.445091520936418,1.33207083179526,0.403563860606914));
#16215=CARTESIAN_POINT('Ctrl Pts',(0.484488022261586,1.30643330531434,0.355304950761552));
#16216=CARTESIAN_POINT('Ctrl Pts',(0.503716463284046,1.3,0.32753749298313));
#16217=CARTESIAN_POINT('Ctrl Pts',(0.53551402125728,1.3,0.27246250701687));
#16218=CARTESIAN_POINT('Ctrl Pts',(0.549947124580676,1.30643330531434,0.241926459727039));
#16219=CARTESIAN_POINT('Ctrl Pts',(0.572042315803119,1.33207083179526,0.183678633836535));
#16220=CARTESIAN_POINT('Ctrl Pts',(0.579820497891285,1.35125503546125,0.15600214762839));
#16221=CARTESIAN_POINT('Ctrl Pts',(0.590063593315144,1.39521815246759,0.111151766652641));
#16222=CARTESIAN_POINT('Ctrl Pts',(0.593243052195919,1.42306587841403,0.0908585874761105));
#16223=CARTESIAN_POINT('Ctrl Pts',(0.596809586309859,1.48451833822352,0.0633319361811906));
#16224=CARTESIAN_POINT('Ctrl Pts',(0.59736109069228,1.51816397144501,0.0562114519197835));
#16225=CARTESIAN_POINT('Ctrl Pts',(0.59736109069228,1.55,0.0562114519197835));
#16226=CARTESIAN_POINT('Origin',(0.,1.55,0.));
#16227=CARTESIAN_POINT('',(-0.347361090692279,1.55,-0.489224153812003));
#16228=CARTESIAN_POINT('Ctrl Pts',(-0.347361090692279,1.55,-0.489224153812003));
#16229=CARTESIAN_POINT('Ctrl Pts',(-0.347361090692279,1.51816397144501,
-0.489224153812003));
#16230=CARTESIAN_POINT('Ctrl Pts',(-0.353251858758695,1.48451833822352,
-0.485186294875824));
#16231=CARTESIAN_POINT('Ctrl Pts',(-0.375307371004241,1.42306587841403,
-0.468334260082228));
#16232=CARTESIAN_POINT('Ctrl Pts',(-0.391292050254278,1.39521815246759,
-0.455434178332924));
#16233=CARTESIAN_POINT('Ctrl Pts',(-0.425012071836758,1.35125503546125,
-0.4241382069946));
#16234=CARTESIAN_POINT('Ctrl Pts',(-0.445091520936419,1.33207083179526,
-0.403563860606914));
#16235=CARTESIAN_POINT('Ctrl Pts',(-0.484488022261586,1.30643330531434,
-0.355304950761552));
#16236=CARTESIAN_POINT('Ctrl Pts',(-0.503716463284046,1.3,-0.32753749298313));
#16237=CARTESIAN_POINT('Ctrl Pts',(-0.53551402125728,1.3,-0.27246250701687));
#16238=CARTESIAN_POINT('Ctrl Pts',(-0.549947124580676,1.30643330531434,
-0.241926459727039));
#16239=CARTESIAN_POINT('Ctrl Pts',(-0.572042315803119,1.33207083179526,
-0.183678633836535));
#16240=CARTESIAN_POINT('Ctrl Pts',(-0.579820497891285,1.35125503546125,
-0.15600214762839));
#16241=CARTESIAN_POINT('Ctrl Pts',(-0.590063593315144,1.39521815246759,
-0.111151766652641));
#16242=CARTESIAN_POINT('Ctrl Pts',(-0.593243052195918,1.42306587841403,
-0.0908585874761106));
#16243=CARTESIAN_POINT('Ctrl Pts',(-0.596809586309859,1.48451833822352,
-0.0633319361811906));
#16244=CARTESIAN_POINT('Ctrl Pts',(-0.597361090692279,1.51816397144501,
-0.0562114519197835));
#16245=CARTESIAN_POINT('Ctrl Pts',(-0.597361090692279,1.58183602855499,
-0.0562114519197835));
#16246=CARTESIAN_POINT('Ctrl Pts',(-0.596809586309859,1.61548166177647,
-0.0633319361811905));
#16247=CARTESIAN_POINT('Ctrl Pts',(-0.593243052195918,1.67693412158597,
-0.0908585874761104));
#16248=CARTESIAN_POINT('Ctrl Pts',(-0.590063593315144,1.70478184753241,
-0.111151766652641));
#16249=CARTESIAN_POINT('Ctrl Pts',(-0.579820497891285,1.74874496453875,
-0.15600214762839));
#16250=CARTESIAN_POINT('Ctrl Pts',(-0.572042315803118,1.76792916820474,
-0.183678633836535));
#16251=CARTESIAN_POINT('Ctrl Pts',(-0.549947124580676,1.79356669468566,
-0.241926459727039));
#16252=CARTESIAN_POINT('Ctrl Pts',(-0.53551402125728,1.8,-0.27246250701687));
#16253=CARTESIAN_POINT('Ctrl Pts',(-0.503716463284046,1.8,-0.32753749298313));
#16254=CARTESIAN_POINT('Ctrl Pts',(-0.484488022261586,1.79356669468566,
-0.355304950761552));
#16255=CARTESIAN_POINT('Ctrl Pts',(-0.445091520936419,1.76792916820474,
-0.403563860606914));
#16256=CARTESIAN_POINT('Ctrl Pts',(-0.425012071836758,1.74874496453875,
-0.4241382069946));
#16257=CARTESIAN_POINT('Ctrl Pts',(-0.391292050254278,1.70478184753241,
-0.455434178332924));
#16258=CARTESIAN_POINT('Ctrl Pts',(-0.375307371004241,1.67693412158597,
-0.468334260082228));
#16259=CARTESIAN_POINT('Ctrl Pts',(-0.353251858758695,1.61548166177648,
-0.485186294875824));
#16260=CARTESIAN_POINT('Ctrl Pts',(-0.347361090692279,1.58183602855499,
-0.489224153812003));
#16261=CARTESIAN_POINT('Ctrl Pts',(-0.347361090692279,1.55,-0.489224153812003));
#16262=CARTESIAN_POINT('',(-1.28744468918255,1.55,-1.03198167246111));
#16263=CARTESIAN_POINT('',(0.125,1.55,-0.21650635094611));
#16264=CARTESIAN_POINT('',(-1.42894191624432,1.3,-0.825000000000001));
#16265=CARTESIAN_POINT('Ctrl Pts',(-1.42894191624432,1.3,-0.825000000000001));
#16266=CARTESIAN_POINT('Ctrl Pts',(-1.4132207435299,1.3,-0.852229869895949));
#16267=CARTESIAN_POINT('Ctrl Pts',(-1.39561049050871,1.30629366210296,-0.880751161609749));
#16268=CARTESIAN_POINT('Ctrl Pts',(-1.36172049302549,1.33182222741682,-0.932292094146256));
#16269=CARTESIAN_POINT('Ctrl Pts',(-1.34548213209931,1.35105447038507,-0.955340251466735));
#16270=CARTESIAN_POINT('Ctrl Pts',(-1.31917543061769,1.39539254159618,-0.991349264982991));
#16271=CARTESIAN_POINT('Ctrl Pts',(-1.30734972067592,1.42347183818157,-1.00672880483252));
#16272=CARTESIAN_POINT('Ctrl Pts',(-1.29146042158868,1.48505200040818,-1.02703269653942));
#16273=CARTESIAN_POINT('Ctrl Pts',(-1.28744468918255,1.51855708359447,-1.03198167246111));
#16274=CARTESIAN_POINT('Ctrl Pts',(-1.28744468918255,1.55,-1.03198167246111));
#16275=CARTESIAN_POINT('',(-1.42894191624432,1.8,-0.825000000000001));
#16276=CARTESIAN_POINT('Ctrl Pts',(-1.42894191624432,1.8,-0.825000000000001));
#16277=CARTESIAN_POINT('Ctrl Pts',(-1.44466308895875,1.8,-0.797770130104052));
#16278=CARTESIAN_POINT('Ctrl Pts',(-1.46055812562105,1.79370633789704,-0.768258557763732));
#16279=CARTESIAN_POINT('Ctrl Pts',(-1.48824888379079,1.76817777258318,-0.713138492740816));
#16280=CARTESIAN_POINT('Ctrl Pts',(-1.50008999307766,1.74894552961493,-0.687551581002689));
#16281=CARTESIAN_POINT('Ctrl Pts',(-1.51812136280714,1.70460745840382,-0.646764802471699));
#16282=CARTESIAN_POINT('Ctrl Pts',(-1.52552758004446,1.67652816181843,-0.628833667319578));
#16283=CARTESIAN_POINT('Ctrl Pts',(-1.53516661651472,1.61494799959182,-0.60492118480825));
#16284=CARTESIAN_POINT('Ctrl Pts',(-1.53744468918255,1.58144291640553,-0.598968970568896));
#16285=CARTESIAN_POINT('Ctrl Pts',(-1.53744468918255,1.51855708359447,-0.598968970568896));
#16286=CARTESIAN_POINT('Ctrl Pts',(-1.53516661651472,1.48505200040818,-0.60492118480825));
#16287=CARTESIAN_POINT('Ctrl Pts',(-1.52552758004446,1.42347183818157,-0.628833667319578));
#16288=CARTESIAN_POINT('Ctrl Pts',(-1.51812136280714,1.39539254159618,-0.646764802471699));
#16289=CARTESIAN_POINT('Ctrl Pts',(-1.50008999307766,1.35105447038507,-0.687551581002689));
#16290=CARTESIAN_POINT('Ctrl Pts',(-1.48824888379079,1.33182222741682,-0.713138492740816));
#16291=CARTESIAN_POINT('Ctrl Pts',(-1.46055812562105,1.30629366210296,-0.768258557763732));
#16292=CARTESIAN_POINT('Ctrl Pts',(-1.44466308895875,1.3,-0.797770130104052));
#16293=CARTESIAN_POINT('Ctrl Pts',(-1.42894191624432,1.3,-0.825000000000001));
#16294=CARTESIAN_POINT('Ctrl Pts',(-1.28744468918255,1.55,-1.03198167246111));
#16295=CARTESIAN_POINT('Ctrl Pts',(-1.28744468918255,1.58144291640553,-1.03198167246111));
#16296=CARTESIAN_POINT('Ctrl Pts',(-1.29146042158868,1.61494799959182,-1.02703269653942));
#16297=CARTESIAN_POINT('Ctrl Pts',(-1.30734972067592,1.67652816181843,-1.00672880483252));
#16298=CARTESIAN_POINT('Ctrl Pts',(-1.31917543061769,1.70460745840382,-0.991349264982991));
#16299=CARTESIAN_POINT('Ctrl Pts',(-1.34548213209931,1.74894552961493,-0.955340251466734));
#16300=CARTESIAN_POINT('Ctrl Pts',(-1.36172049302549,1.76817777258318,-0.932292094146256));
#16301=CARTESIAN_POINT('Ctrl Pts',(-1.39561049050871,1.79370633789704,-0.880751161609749));
#16302=CARTESIAN_POINT('Ctrl Pts',(-1.4132207435299,1.8,-0.852229869895949));
#16303=CARTESIAN_POINT('Ctrl Pts',(-1.42894191624432,1.8,-0.825000000000001));
#16304=CARTESIAN_POINT('Origin',(0.,1.55,0.));
#16305=CARTESIAN_POINT('',(-1.65,0.85,-2.02066721859313E-16));
#16306=CARTESIAN_POINT('Origin',(0.,0.85,0.));
#16307=CARTESIAN_POINT('',(-1.65,2.25,-2.02066721859313E-16));
#16308=CARTESIAN_POINT('',(-1.65,1.55,-2.02066721859313E-16));
#16309=CARTESIAN_POINT('Origin',(0.,2.25,0.));
#16310=CARTESIAN_POINT('',(-1.42894191624432,1.3,0.825));
#16311=CARTESIAN_POINT('',(-1.42894191624432,1.8,0.825));
#16312=CARTESIAN_POINT('Ctrl Pts',(-1.42894191624432,1.3,0.825));
#16313=CARTESIAN_POINT('Ctrl Pts',(-1.44466308895875,1.3,0.797770130104051));
#16314=CARTESIAN_POINT('Ctrl Pts',(-1.46055812562105,1.30629366210296,0.768258557763731));
#16315=CARTESIAN_POINT('Ctrl Pts',(-1.48824888379079,1.33182222741682,0.713138492740815));
#16316=CARTESIAN_POINT('Ctrl Pts',(-1.50008999307766,1.35105447038507,0.687551581002688));
#16317=CARTESIAN_POINT('Ctrl Pts',(-1.51812136280714,1.39539254159618,0.646764802471698));
#16318=CARTESIAN_POINT('Ctrl Pts',(-1.52552758004446,1.42347183818157,0.628833667319577));
#16319=CARTESIAN_POINT('Ctrl Pts',(-1.53516661651472,1.48505200040818,0.604921184808249));
#16320=CARTESIAN_POINT('Ctrl Pts',(-1.53744468918255,1.51855708359447,0.598968970568895));
#16321=CARTESIAN_POINT('Ctrl Pts',(-1.53744468918255,1.58144291640553,0.598968970568895));
#16322=CARTESIAN_POINT('Ctrl Pts',(-1.53516661651472,1.61494799959182,0.604921184808249));
#16323=CARTESIAN_POINT('Ctrl Pts',(-1.52552758004446,1.67652816181843,0.628833667319577));
#16324=CARTESIAN_POINT('Ctrl Pts',(-1.51812136280714,1.70460745840382,0.646764802471698));
#16325=CARTESIAN_POINT('Ctrl Pts',(-1.50008999307766,1.74894552961493,0.687551581002688));
#16326=CARTESIAN_POINT('Ctrl Pts',(-1.48824888379079,1.76817777258318,0.713138492740815));
#16327=CARTESIAN_POINT('Ctrl Pts',(-1.46055812562105,1.79370633789704,0.768258557763731));
#16328=CARTESIAN_POINT('Ctrl Pts',(-1.44466308895875,1.8,0.797770130104051));
#16329=CARTESIAN_POINT('Ctrl Pts',(-1.42894191624432,1.8,0.825));
#16330=CARTESIAN_POINT('',(-1.28744468918255,1.55,1.03198167246111));
#16331=CARTESIAN_POINT('Ctrl Pts',(-1.42894191624432,1.8,0.825));
#16332=CARTESIAN_POINT('Ctrl Pts',(-1.4132207435299,1.8,0.852229869895948));
#16333=CARTESIAN_POINT('Ctrl Pts',(-1.39561049050871,1.79370633789704,0.880751161609747));
#16334=CARTESIAN_POINT('Ctrl Pts',(-1.36172049302549,1.76817777258318,0.932292094146255));
#16335=CARTESIAN_POINT('Ctrl Pts',(-1.34548213209931,1.74894552961493,0.955340251466733));
#16336=CARTESIAN_POINT('Ctrl Pts',(-1.31917543061769,1.70460745840382,0.991349264982989));
#16337=CARTESIAN_POINT('Ctrl Pts',(-1.30734972067592,1.67652816181843,1.00672880483252));
#16338=CARTESIAN_POINT('Ctrl Pts',(-1.29146042158868,1.61494799959182,1.02703269653942));
#16339=CARTESIAN_POINT('Ctrl Pts',(-1.28744468918255,1.58144291640553,1.03198167246111));
#16340=CARTESIAN_POINT('Ctrl Pts',(-1.28744468918255,1.55,1.03198167246111));
#16341=CARTESIAN_POINT('Ctrl Pts',(-1.28744468918255,1.55,1.03198167246111));
#16342=CARTESIAN_POINT('Ctrl Pts',(-1.28744468918255,1.51855708359447,1.03198167246111));
#16343=CARTESIAN_POINT('Ctrl Pts',(-1.29146042158868,1.48505200040818,1.02703269653942));
#16344=CARTESIAN_POINT('Ctrl Pts',(-1.30734972067592,1.42347183818157,1.00672880483252));
#16345=CARTESIAN_POINT('Ctrl Pts',(-1.31917543061769,1.39539254159618,0.99134926498299));
#16346=CARTESIAN_POINT('Ctrl Pts',(-1.34548213209931,1.35105447038508,0.955340251466733));
#16347=CARTESIAN_POINT('Ctrl Pts',(-1.36172049302549,1.33182222741682,0.932292094146255));
#16348=CARTESIAN_POINT('Ctrl Pts',(-1.39561049050871,1.30629366210296,0.880751161609748));
#16349=CARTESIAN_POINT('Ctrl Pts',(-1.4132207435299,1.3,0.852229869895949));
#16350=CARTESIAN_POINT('Ctrl Pts',(-1.42894191624432,1.3,0.825));
#16351=CARTESIAN_POINT('',(1.42894191624432,1.8,-0.825));
#16352=CARTESIAN_POINT('',(1.42894191624432,1.3,-0.825));
#16353=CARTESIAN_POINT('Ctrl Pts',(1.42894191624432,1.8,-0.825));
#16354=CARTESIAN_POINT('Ctrl Pts',(1.4132207435299,1.8,-0.852229869895949));
#16355=CARTESIAN_POINT('Ctrl Pts',(1.39561049050871,1.79370633789704,-0.880751161609748));
#16356=CARTESIAN_POINT('Ctrl Pts',(1.36172049302549,1.76817777258318,-0.932292094146255));
#16357=CARTESIAN_POINT('Ctrl Pts',(1.34548213209931,1.74894552961493,-0.955340251466734));
#16358=CARTESIAN_POINT('Ctrl Pts',(1.31917543061769,1.70460745840382,-0.99134926498299));
#16359=CARTESIAN_POINT('Ctrl Pts',(1.30734972067592,1.67652816181843,-1.00672880483252));
#16360=CARTESIAN_POINT('Ctrl Pts',(1.29146042158868,1.61494799959182,-1.02703269653942));
#16361=CARTESIAN_POINT('Ctrl Pts',(1.28744468918255,1.58144291640553,-1.03198167246111));
#16362=CARTESIAN_POINT('Ctrl Pts',(1.28744468918255,1.51855708359447,-1.03198167246111));
#16363=CARTESIAN_POINT('Ctrl Pts',(1.29146042158868,1.48505200040818,-1.02703269653942));
#16364=CARTESIAN_POINT('Ctrl Pts',(1.30734972067592,1.42347183818157,-1.00672880483252));
#16365=CARTESIAN_POINT('Ctrl Pts',(1.31917543061769,1.39539254159618,-0.99134926498299));
#16366=CARTESIAN_POINT('Ctrl Pts',(1.34548213209931,1.35105447038507,-0.955340251466734));
#16367=CARTESIAN_POINT('Ctrl Pts',(1.36172049302549,1.33182222741682,-0.932292094146255));
#16368=CARTESIAN_POINT('Ctrl Pts',(1.39561049050871,1.30629366210296,-0.880751161609748));
#16369=CARTESIAN_POINT('Ctrl Pts',(1.4132207435299,1.3,-0.852229869895948));
#16370=CARTESIAN_POINT('Ctrl Pts',(1.42894191624432,1.3,-0.825));
#16371=CARTESIAN_POINT('',(1.53744468918255,1.55,-0.598968970568895));
#16372=CARTESIAN_POINT('Ctrl Pts',(1.42894191624432,1.3,-0.825));
#16373=CARTESIAN_POINT('Ctrl Pts',(1.44466308895875,1.3,-0.797770130104051));
#16374=CARTESIAN_POINT('Ctrl Pts',(1.46055812562105,1.30629366210296,-0.768258557763731));
#16375=CARTESIAN_POINT('Ctrl Pts',(1.48824888379079,1.33182222741682,-0.713138492740815));
#16376=CARTESIAN_POINT('Ctrl Pts',(1.50008999307766,1.35105447038507,-0.687551581002688));
#16377=CARTESIAN_POINT('Ctrl Pts',(1.51812136280714,1.39539254159618,-0.646764802471698));
#16378=CARTESIAN_POINT('Ctrl Pts',(1.52552758004446,1.42347183818157,-0.628833667319577));
#16379=CARTESIAN_POINT('Ctrl Pts',(1.53516661651472,1.48505200040818,-0.604921184808249));
#16380=CARTESIAN_POINT('Ctrl Pts',(1.53744468918255,1.51855708359447,-0.598968970568895));
#16381=CARTESIAN_POINT('Ctrl Pts',(1.53744468918255,1.55,-0.598968970568895));
#16382=CARTESIAN_POINT('Ctrl Pts',(1.53744468918255,1.55,-0.598968970568895));
#16383=CARTESIAN_POINT('Ctrl Pts',(1.53744468918255,1.58144291640553,-0.598968970568895));
#16384=CARTESIAN_POINT('Ctrl Pts',(1.53516661651472,1.61494799959182,-0.604921184808249));
#16385=CARTESIAN_POINT('Ctrl Pts',(1.52552758004446,1.67652816181843,-0.628833667319577));
#16386=CARTESIAN_POINT('Ctrl Pts',(1.51812136280714,1.70460745840382,-0.646764802471698));
#16387=CARTESIAN_POINT('Ctrl Pts',(1.50008999307766,1.74894552961493,-0.687551581002688));
#16388=CARTESIAN_POINT('Ctrl Pts',(1.48824888379079,1.76817777258318,-0.713138492740815));
#16389=CARTESIAN_POINT('Ctrl Pts',(1.46055812562105,1.79370633789704,-0.768258557763731));
#16390=CARTESIAN_POINT('Ctrl Pts',(1.44466308895875,1.8,-0.797770130104051));
#16391=CARTESIAN_POINT('Ctrl Pts',(1.42894191624432,1.8,-0.825));
#16392=CARTESIAN_POINT('',(0.,1.3,-1.65));
#16393=CARTESIAN_POINT('',(0.,1.8,-1.65));
#16394=CARTESIAN_POINT('Ctrl Pts',(1.38777878078145E-17,1.3,-1.65));
#16395=CARTESIAN_POINT('Ctrl Pts',(0.0314423454288489,1.3,-1.65));
#16396=CARTESIAN_POINT('Ctrl Pts',(0.0649476351123396,1.30629366210296,
-1.64900971937348));
#16397=CARTESIAN_POINT('Ctrl Pts',(0.126528390765307,1.33182222741682,-1.64543058688707));
#16398=CARTESIAN_POINT('Ctrl Pts',(0.154607860978348,1.35105447038507,-1.64289183246942));
#16399=CARTESIAN_POINT('Ctrl Pts',(0.198945932189457,1.39539254159618,-1.63811406745469));
#16400=CARTESIAN_POINT('Ctrl Pts',(0.218177859368546,1.42347183818157,-1.63556247215209));
#16401=CARTESIAN_POINT('Ctrl Pts',(0.243706194926033,1.48505200040818,-1.63195388134767));
#16402=CARTESIAN_POINT('Ctrl Pts',(0.25,1.51855708359447,-1.63095064303001));
#16403=CARTESIAN_POINT('Ctrl Pts',(0.25,1.58144291640553,-1.63095064303001));
#16404=CARTESIAN_POINT('Ctrl Pts',(0.243706194926033,1.61494799959182,-1.63195388134767));
#16405=CARTESIAN_POINT('Ctrl Pts',(0.218177859368546,1.67652816181843,-1.63556247215209));
#16406=CARTESIAN_POINT('Ctrl Pts',(0.198945932189457,1.70460745840382,-1.63811406745469));
#16407=CARTESIAN_POINT('Ctrl Pts',(0.154607860978349,1.74894552961493,-1.64289183246942));
#16408=CARTESIAN_POINT('Ctrl Pts',(0.126528390765307,1.76817777258318,-1.64543058688707));
#16409=CARTESIAN_POINT('Ctrl Pts',(0.0649476351123398,1.79370633789704,
-1.64900971937348));
#16410=CARTESIAN_POINT('Ctrl Pts',(0.031442345428849,1.8,-1.65));
#16411=CARTESIAN_POINT('Ctrl Pts',(7.63278329429795E-17,1.8,-1.65));
#16412=CARTESIAN_POINT('',(-0.25,1.55,-1.63095064303001));
#16413=CARTESIAN_POINT('Ctrl Pts',(9.0205620750794E-17,1.8,-1.65));
#16414=CARTESIAN_POINT('Ctrl Pts',(-0.0314423454288488,1.8,-1.65));
#16415=CARTESIAN_POINT('Ctrl Pts',(-0.0649476351123396,1.79370633789704,
-1.64900971937348));
#16416=CARTESIAN_POINT('Ctrl Pts',(-0.126528390765307,1.76817777258318,
-1.64543058688707));
#16417=CARTESIAN_POINT('Ctrl Pts',(-0.154607860978348,1.74894552961493,
-1.64289183246942));
#16418=CARTESIAN_POINT('Ctrl Pts',(-0.198945932189456,1.70460745840382,
-1.63811406745469));
#16419=CARTESIAN_POINT('Ctrl Pts',(-0.218177859368546,1.67652816181843,
-1.63556247215209));
#16420=CARTESIAN_POINT('Ctrl Pts',(-0.243706194926033,1.61494799959182,
-1.63195388134767));
#16421=CARTESIAN_POINT('Ctrl Pts',(-0.25,1.58144291640553,-1.63095064303001));
#16422=CARTESIAN_POINT('Ctrl Pts',(-0.25,1.55,-1.63095064303001));
#16423=CARTESIAN_POINT('Ctrl Pts',(-0.25,1.55,-1.63095064303001));
#16424=CARTESIAN_POINT('Ctrl Pts',(-0.25,1.51855708359447,-1.63095064303001));
#16425=CARTESIAN_POINT('Ctrl Pts',(-0.243706194926033,1.48505200040818,
-1.63195388134767));
#16426=CARTESIAN_POINT('Ctrl Pts',(-0.218177859368546,1.42347183818157,
-1.63556247215209));
#16427=CARTESIAN_POINT('Ctrl Pts',(-0.198945932189457,1.39539254159618,
-1.63811406745469));
#16428=CARTESIAN_POINT('Ctrl Pts',(-0.154607860978349,1.35105447038507,
-1.64289183246942));
#16429=CARTESIAN_POINT('Ctrl Pts',(-0.126528390765307,1.33182222741682,
-1.64543058688707));
#16430=CARTESIAN_POINT('Ctrl Pts',(-0.0649476351123398,1.30629366210296,
-1.64900971937348));
#16431=CARTESIAN_POINT('Ctrl Pts',(-0.031442345428849,1.3,-1.65));
#16432=CARTESIAN_POINT('Ctrl Pts',(-4.85722573273506E-17,1.3,-1.65));
#16433=CARTESIAN_POINT('',(0.,1.8,1.65));
#16434=CARTESIAN_POINT('',(0.,1.3,1.65));
#16435=CARTESIAN_POINT('Ctrl Pts',(8.32667268468867E-17,1.8,1.65));
#16436=CARTESIAN_POINT('Ctrl Pts',(0.031442345428849,1.8,1.65));
#16437=CARTESIAN_POINT('Ctrl Pts',(0.0649476351123398,1.79370633789704,
1.64900971937348));
#16438=CARTESIAN_POINT('Ctrl Pts',(0.126528390765307,1.76817777258318,1.64543058688707));
#16439=CARTESIAN_POINT('Ctrl Pts',(0.154607860978349,1.74894552961493,1.64289183246942));
#16440=CARTESIAN_POINT('Ctrl Pts',(0.198945932189457,1.70460745840382,1.63811406745469));
#16441=CARTESIAN_POINT('Ctrl Pts',(0.218177859368546,1.67652816181843,1.63556247215209));
#16442=CARTESIAN_POINT('Ctrl Pts',(0.243706194926033,1.61494799959182,1.63195388134767));
#16443=CARTESIAN_POINT('Ctrl Pts',(0.25,1.58144291640553,1.63095064303001));
#16444=CARTESIAN_POINT('Ctrl Pts',(0.25,1.51855708359447,1.63095064303001));
#16445=CARTESIAN_POINT('Ctrl Pts',(0.243706194926033,1.48505200040818,1.63195388134767));
#16446=CARTESIAN_POINT('Ctrl Pts',(0.218177859368546,1.42347183818157,1.63556247215209));
#16447=CARTESIAN_POINT('Ctrl Pts',(0.198945932189457,1.39539254159618,1.63811406745469));
#16448=CARTESIAN_POINT('Ctrl Pts',(0.154607860978348,1.35105447038507,1.64289183246942));
#16449=CARTESIAN_POINT('Ctrl Pts',(0.126528390765307,1.33182222741682,1.64543058688707));
#16450=CARTESIAN_POINT('Ctrl Pts',(0.0649476351123397,1.30629366210296,
1.64900971937348));
#16451=CARTESIAN_POINT('Ctrl Pts',(0.0314423454288488,1.3,1.65));
#16452=CARTESIAN_POINT('Ctrl Pts',(-1.38777878078145E-17,1.3,1.65));
#16453=CARTESIAN_POINT('',(-0.25,1.55,1.63095064303001));
#16454=CARTESIAN_POINT('Ctrl Pts',(-5.55111512312578E-17,1.3,1.65));
#16455=CARTESIAN_POINT('Ctrl Pts',(-0.031442345428849,1.3,1.65));
#16456=CARTESIAN_POINT('Ctrl Pts',(-0.0649476351123398,1.30629366210296,
1.64900971937348));
#16457=CARTESIAN_POINT('Ctrl Pts',(-0.126528390765307,1.33182222741682,
1.64543058688707));
#16458=CARTESIAN_POINT('Ctrl Pts',(-0.154607860978349,1.35105447038507,
1.64289183246942));
#16459=CARTESIAN_POINT('Ctrl Pts',(-0.198945932189457,1.39539254159618,
1.63811406745469));
#16460=CARTESIAN_POINT('Ctrl Pts',(-0.218177859368546,1.42347183818157,
1.63556247215209));
#16461=CARTESIAN_POINT('Ctrl Pts',(-0.243706194926033,1.48505200040818,
1.63195388134767));
#16462=CARTESIAN_POINT('Ctrl Pts',(-0.25,1.51855708359447,1.63095064303001));
#16463=CARTESIAN_POINT('Ctrl Pts',(-0.25,1.55,1.63095064303001));
#16464=CARTESIAN_POINT('Ctrl Pts',(-0.25,1.55,1.63095064303001));
#16465=CARTESIAN_POINT('Ctrl Pts',(-0.25,1.58144291640553,1.63095064303001));
#16466=CARTESIAN_POINT('Ctrl Pts',(-0.243706194926033,1.61494799959182,
1.63195388134767));
#16467=CARTESIAN_POINT('Ctrl Pts',(-0.218177859368546,1.67652816181843,
1.63556247215209));
#16468=CARTESIAN_POINT('Ctrl Pts',(-0.198945932189456,1.70460745840382,
1.63811406745469));
#16469=CARTESIAN_POINT('Ctrl Pts',(-0.154607860978348,1.74894552961493,
1.64289183246942));
#16470=CARTESIAN_POINT('Ctrl Pts',(-0.126528390765307,1.76817777258318,
1.64543058688707));
#16471=CARTESIAN_POINT('Ctrl Pts',(-0.0649476351123396,1.79370633789704,
1.64900971937348));
#16472=CARTESIAN_POINT('Ctrl Pts',(-0.0314423454288488,1.8,1.65));
#16473=CARTESIAN_POINT('Ctrl Pts',(7.63278329429795E-17,1.8,1.65));
#16474=CARTESIAN_POINT('Origin',(0.,1.55,0.));
#16475=CARTESIAN_POINT('',(-0.34736109069228,1.55,0.489224153812002));
#16476=CARTESIAN_POINT('',(0.125,1.55,0.21650635094611));
#16477=CARTESIAN_POINT('Ctrl Pts',(-0.34736109069228,1.55,0.489224153812002));
#16478=CARTESIAN_POINT('Ctrl Pts',(-0.34736109069228,1.58183602855499,0.489224153812002));
#16479=CARTESIAN_POINT('Ctrl Pts',(-0.353251858758695,1.61548166177648,
0.485186294875824));
#16480=CARTESIAN_POINT('Ctrl Pts',(-0.375307371004242,1.67693412158597,
0.468334260082228));
#16481=CARTESIAN_POINT('Ctrl Pts',(-0.391292050254279,1.70478184753241,
0.455434178332924));
#16482=CARTESIAN_POINT('Ctrl Pts',(-0.425012071836758,1.74874496453875,
0.424138206994599));
#16483=CARTESIAN_POINT('Ctrl Pts',(-0.445091520936419,1.76792916820474,
0.403563860606914));
#16484=CARTESIAN_POINT('Ctrl Pts',(-0.484488022261587,1.79356669468566,
0.355304950761552));
#16485=CARTESIAN_POINT('Ctrl Pts',(-0.503716463284046,1.8,0.32753749298313));
#16486=CARTESIAN_POINT('Ctrl Pts',(-0.535514021257281,1.8,0.27246250701687));
#16487=CARTESIAN_POINT('Ctrl Pts',(-0.549947124580677,1.79356669468566,
0.241926459727038));
#16488=CARTESIAN_POINT('Ctrl Pts',(-0.572042315803119,1.76792916820474,
0.183678633836535));
#16489=CARTESIAN_POINT('Ctrl Pts',(-0.579820497891285,1.74874496453875,
0.156002147628389));
#16490=CARTESIAN_POINT('Ctrl Pts',(-0.590063593315144,1.70478184753241,
0.11115176665264));
#16491=CARTESIAN_POINT('Ctrl Pts',(-0.593243052195919,1.67693412158597,
0.0908585874761102));
#16492=CARTESIAN_POINT('Ctrl Pts',(-0.596809586309859,1.61548166177648,
0.0633319361811903));
#16493=CARTESIAN_POINT('Ctrl Pts',(-0.59736109069228,1.58183602855499,0.0562114519197831));
#16494=CARTESIAN_POINT('Ctrl Pts',(-0.59736109069228,1.51816397144501,0.0562114519197831));
#16495=CARTESIAN_POINT('Ctrl Pts',(-0.596809586309859,1.48451833822352,
0.0633319361811902));
#16496=CARTESIAN_POINT('Ctrl Pts',(-0.593243052195919,1.42306587841403,
0.0908585874761101));
#16497=CARTESIAN_POINT('Ctrl Pts',(-0.590063593315144,1.39521815246759,
0.11115176665264));
#16498=CARTESIAN_POINT('Ctrl Pts',(-0.579820497891285,1.35125503546125,
0.156002147628389));
#16499=CARTESIAN_POINT('Ctrl Pts',(-0.572042315803119,1.33207083179526,
0.183678633836535));
#16500=CARTESIAN_POINT('Ctrl Pts',(-0.549947124580676,1.30643330531434,
0.241926459727038));
#16501=CARTESIAN_POINT('Ctrl Pts',(-0.535514021257281,1.3,0.27246250701687));
#16502=CARTESIAN_POINT('Ctrl Pts',(-0.503716463284046,1.3,0.32753749298313));
#16503=CARTESIAN_POINT('Ctrl Pts',(-0.484488022261587,1.30643330531434,
0.355304950761552));
#16504=CARTESIAN_POINT('Ctrl Pts',(-0.445091520936419,1.33207083179526,
0.403563860606914));
#16505=CARTESIAN_POINT('Ctrl Pts',(-0.425012071836758,1.35125503546125,
0.424138206994599));
#16506=CARTESIAN_POINT('Ctrl Pts',(-0.391292050254279,1.39521815246759,
0.455434178332924));
#16507=CARTESIAN_POINT('Ctrl Pts',(-0.375307371004241,1.42306587841403,
0.468334260082228));
#16508=CARTESIAN_POINT('Ctrl Pts',(-0.353251858758695,1.48451833822352,
0.485186294875824));
#16509=CARTESIAN_POINT('Ctrl Pts',(-0.34736109069228,1.51816397144501,0.489224153812002));
#16510=CARTESIAN_POINT('Ctrl Pts',(-0.34736109069228,1.55,0.489224153812002));
#16511=CARTESIAN_POINT('Origin',(0.,1.55,0.));
#16512=CARTESIAN_POINT('',(0.59736109069228,1.55,-0.0562114519197831));
#16513=CARTESIAN_POINT('Ctrl Pts',(0.59736109069228,1.55,-0.0562114519197831));
#16514=CARTESIAN_POINT('Ctrl Pts',(0.59736109069228,1.51816397144501,-0.0562114519197831));
#16515=CARTESIAN_POINT('Ctrl Pts',(0.596809586309859,1.48451833822352,-0.0633319361811902));
#16516=CARTESIAN_POINT('Ctrl Pts',(0.593243052195919,1.42306587841403,-0.0908585874761101));
#16517=CARTESIAN_POINT('Ctrl Pts',(0.590063593315144,1.39521815246759,-0.11115176665264));
#16518=CARTESIAN_POINT('Ctrl Pts',(0.579820497891285,1.35125503546125,-0.156002147628389));
#16519=CARTESIAN_POINT('Ctrl Pts',(0.572042315803119,1.33207083179526,-0.183678633836535));
#16520=CARTESIAN_POINT('Ctrl Pts',(0.549947124580677,1.30643330531434,-0.241926459727038));
#16521=CARTESIAN_POINT('Ctrl Pts',(0.535514021257281,1.3,-0.27246250701687));
#16522=CARTESIAN_POINT('Ctrl Pts',(0.503716463284046,1.3,-0.32753749298313));
#16523=CARTESIAN_POINT('Ctrl Pts',(0.484488022261587,1.30643330531434,-0.355304950761552));
#16524=CARTESIAN_POINT('Ctrl Pts',(0.445091520936419,1.33207083179526,-0.403563860606914));
#16525=CARTESIAN_POINT('Ctrl Pts',(0.425012071836758,1.35125503546125,-0.424138206994599));
#16526=CARTESIAN_POINT('Ctrl Pts',(0.391292050254279,1.39521815246759,-0.455434178332924));
#16527=CARTESIAN_POINT('Ctrl Pts',(0.375307371004241,1.42306587841403,-0.468334260082228));
#16528=CARTESIAN_POINT('Ctrl Pts',(0.353251858758695,1.48451833822352,-0.485186294875824));
#16529=CARTESIAN_POINT('Ctrl Pts',(0.34736109069228,1.51816397144501,-0.489224153812002));
#16530=CARTESIAN_POINT('Ctrl Pts',(0.34736109069228,1.58183602855499,-0.489224153812002));
#16531=CARTESIAN_POINT('Ctrl Pts',(0.353251858758695,1.61548166177647,-0.485186294875824));
#16532=CARTESIAN_POINT('Ctrl Pts',(0.375307371004241,1.67693412158597,-0.468334260082228));
#16533=CARTESIAN_POINT('Ctrl Pts',(0.391292050254279,1.70478184753241,-0.455434178332924));
#16534=CARTESIAN_POINT('Ctrl Pts',(0.425012071836758,1.74874496453875,-0.424138206994599));
#16535=CARTESIAN_POINT('Ctrl Pts',(0.445091520936419,1.76792916820474,-0.403563860606914));
#16536=CARTESIAN_POINT('Ctrl Pts',(0.484488022261587,1.79356669468566,-0.355304950761552));
#16537=CARTESIAN_POINT('Ctrl Pts',(0.503716463284046,1.8,-0.32753749298313));
#16538=CARTESIAN_POINT('Ctrl Pts',(0.535514021257281,1.8,-0.27246250701687));
#16539=CARTESIAN_POINT('Ctrl Pts',(0.549947124580677,1.79356669468566,-0.241926459727038));
#16540=CARTESIAN_POINT('Ctrl Pts',(0.572042315803119,1.76792916820474,-0.183678633836535));
#16541=CARTESIAN_POINT('Ctrl Pts',(0.579820497891285,1.74874496453875,-0.156002147628389));
#16542=CARTESIAN_POINT('Ctrl Pts',(0.590063593315144,1.70478184753241,-0.111151766652641));
#16543=CARTESIAN_POINT('Ctrl Pts',(0.593243052195919,1.67693412158597,-0.0908585874761104));
#16544=CARTESIAN_POINT('Ctrl Pts',(0.596809586309859,1.61548166177648,-0.0633319361811903));
#16545=CARTESIAN_POINT('Ctrl Pts',(0.59736109069228,1.58183602855499,-0.0562114519197831));
#16546=CARTESIAN_POINT('Ctrl Pts',(0.59736109069228,1.55,-0.0562114519197831));
#16547=CARTESIAN_POINT('',(0.125,1.55,0.21650635094611));
#16548=CARTESIAN_POINT('Origin',(0.,1.55,0.));
#16549=CARTESIAN_POINT('',(-0.25,1.55,-0.545435605731786));
#16550=CARTESIAN_POINT('',(-0.25,1.55,0.));
#16551=CARTESIAN_POINT('Ctrl Pts',(-0.25,1.55,-0.545435605731786));
#16552=CARTESIAN_POINT('Ctrl Pts',(-0.25,1.58183602855499,-0.545435605731786));
#16553=CARTESIAN_POINT('Ctrl Pts',(-0.243557727551164,1.61548166177648,
-0.548518231057014));
#16554=CARTESIAN_POINT('Ctrl Pts',(-0.217935681191677,1.67693412158597,
-0.559192847558338));
#16555=CARTESIAN_POINT('Ctrl Pts',(-0.198771543060865,1.70478184753241,
-0.566585944985565));
#16556=CARTESIAN_POINT('Ctrl Pts',(-0.154808426054527,1.74874496453875,
-0.580140354622989));
#16557=CARTESIAN_POINT('Ctrl Pts',(-0.1269507948667,1.76792916820474,-0.587242494443449));
#16558=CARTESIAN_POINT('Ctrl Pts',(-0.0654591023190899,1.79356669468566,
-0.597231410488591));
#16559=CARTESIAN_POINT('Ctrl Pts',(-0.0317975579732349,1.8,-0.6));
#16560=CARTESIAN_POINT('Ctrl Pts',(0.0317975579732349,1.8,-0.6));
#16561=CARTESIAN_POINT('Ctrl Pts',(0.0654591023190898,1.79356669468566,
-0.597231410488591));
#16562=CARTESIAN_POINT('Ctrl Pts',(0.1269507948667,1.76792916820474,-0.587242494443449));
#16563=CARTESIAN_POINT('Ctrl Pts',(0.154808426054527,1.74874496453875,-0.580140354622989));
#16564=CARTESIAN_POINT('Ctrl Pts',(0.198771543060865,1.70478184753241,-0.566585944985565));
#16565=CARTESIAN_POINT('Ctrl Pts',(0.217935681191677,1.67693412158597,-0.559192847558338));
#16566=CARTESIAN_POINT('Ctrl Pts',(0.243557727551164,1.61548166177648,-0.548518231057014));
#16567=CARTESIAN_POINT('Ctrl Pts',(0.25,1.58183602855499,-0.545435605731786));
#16568=CARTESIAN_POINT('Ctrl Pts',(0.25,1.51816397144501,-0.545435605731786));
#16569=CARTESIAN_POINT('Ctrl Pts',(0.243557727551164,1.48451833822352,-0.548518231057014));
#16570=CARTESIAN_POINT('Ctrl Pts',(0.217935681191677,1.42306587841403,-0.559192847558338));
#16571=CARTESIAN_POINT('Ctrl Pts',(0.198771543060865,1.39521815246759,-0.566585944985565));
#16572=CARTESIAN_POINT('Ctrl Pts',(0.154808426054527,1.35125503546125,-0.580140354622989));
#16573=CARTESIAN_POINT('Ctrl Pts',(0.1269507948667,1.33207083179526,-0.587242494443449));
#16574=CARTESIAN_POINT('Ctrl Pts',(0.0654591023190899,1.30643330531434,
-0.597231410488591));
#16575=CARTESIAN_POINT('Ctrl Pts',(0.0317975579732349,1.3,-0.6));
#16576=CARTESIAN_POINT('Ctrl Pts',(-0.0317975579732349,1.3,-0.6));
#16577=CARTESIAN_POINT('Ctrl Pts',(-0.0654591023190899,1.30643330531434,
-0.597231410488591));
#16578=CARTESIAN_POINT('Ctrl Pts',(-0.1269507948667,1.33207083179526,-0.587242494443449));
#16579=CARTESIAN_POINT('Ctrl Pts',(-0.154808426054527,1.35125503546125,
-0.580140354622989));
#16580=CARTESIAN_POINT('Ctrl Pts',(-0.198771543060865,1.39521815246759,
-0.566585944985565));
#16581=CARTESIAN_POINT('Ctrl Pts',(-0.217935681191677,1.42306587841403,
-0.559192847558338));
#16582=CARTESIAN_POINT('Ctrl Pts',(-0.243557727551164,1.48451833822352,
-0.548518231057014));
#16583=CARTESIAN_POINT('Ctrl Pts',(-0.25,1.51816397144501,-0.545435605731786));
#16584=CARTESIAN_POINT('Ctrl Pts',(-0.25,1.55,-0.545435605731786));
#16585=CARTESIAN_POINT('Origin',(0.,1.55,0.));
#16586=CARTESIAN_POINT('',(-0.25,1.55,0.545435605731786));
#16587=CARTESIAN_POINT('Ctrl Pts',(-0.25,1.55,0.545435605731786));
#16588=CARTESIAN_POINT('Ctrl Pts',(-0.25,1.51816397144501,0.545435605731786));
#16589=CARTESIAN_POINT('Ctrl Pts',(-0.243557727551164,1.48451833822352,
0.548518231057014));
#16590=CARTESIAN_POINT('Ctrl Pts',(-0.217935681191677,1.42306587841403,
0.559192847558338));
#16591=CARTESIAN_POINT('Ctrl Pts',(-0.198771543060865,1.39521815246759,
0.566585944985565));
#16592=CARTESIAN_POINT('Ctrl Pts',(-0.154808426054527,1.35125503546125,
0.580140354622989));
#16593=CARTESIAN_POINT('Ctrl Pts',(-0.1269507948667,1.33207083179526,0.587242494443449));
#16594=CARTESIAN_POINT('Ctrl Pts',(-0.0654591023190899,1.30643330531434,
0.597231410488591));
#16595=CARTESIAN_POINT('Ctrl Pts',(-0.0317975579732349,1.3,0.6));
#16596=CARTESIAN_POINT('Ctrl Pts',(0.0317975579732349,1.3,0.6));
#16597=CARTESIAN_POINT('Ctrl Pts',(0.0654591023190899,1.30643330531434,
0.597231410488591));
#16598=CARTESIAN_POINT('Ctrl Pts',(0.1269507948667,1.33207083179526,0.587242494443449));
#16599=CARTESIAN_POINT('Ctrl Pts',(0.154808426054527,1.35125503546125,0.580140354622989));
#16600=CARTESIAN_POINT('Ctrl Pts',(0.198771543060865,1.39521815246759,0.566585944985565));
#16601=CARTESIAN_POINT('Ctrl Pts',(0.217935681191677,1.42306587841403,0.559192847558338));
#16602=CARTESIAN_POINT('Ctrl Pts',(0.243557727551164,1.48451833822352,0.548518231057014));
#16603=CARTESIAN_POINT('Ctrl Pts',(0.25,1.51816397144501,0.545435605731786));
#16604=CARTESIAN_POINT('Ctrl Pts',(0.25,1.58183602855499,0.545435605731786));
#16605=CARTESIAN_POINT('Ctrl Pts',(0.243557727551164,1.61548166177648,0.548518231057014));
#16606=CARTESIAN_POINT('Ctrl Pts',(0.217935681191677,1.67693412158597,0.559192847558338));
#16607=CARTESIAN_POINT('Ctrl Pts',(0.198771543060865,1.70478184753241,0.566585944985565));
#16608=CARTESIAN_POINT('Ctrl Pts',(0.154808426054527,1.74874496453875,0.580140354622989));
#16609=CARTESIAN_POINT('Ctrl Pts',(0.1269507948667,1.76792916820474,0.587242494443449));
#16610=CARTESIAN_POINT('Ctrl Pts',(0.0654591023190898,1.79356669468566,
0.597231410488591));
#16611=CARTESIAN_POINT('Ctrl Pts',(0.0317975579732349,1.8,0.6));
#16612=CARTESIAN_POINT('Ctrl Pts',(-0.0317975579732349,1.8,0.6));
#16613=CARTESIAN_POINT('Ctrl Pts',(-0.0654591023190898,1.79356669468566,
0.597231410488591));
#16614=CARTESIAN_POINT('Ctrl Pts',(-0.1269507948667,1.76792916820474,0.587242494443449));
#16615=CARTESIAN_POINT('Ctrl Pts',(-0.154808426054527,1.74874496453875,
0.580140354622989));
#16616=CARTESIAN_POINT('Ctrl Pts',(-0.198771543060865,1.70478184753241,
0.566585944985565));
#16617=CARTESIAN_POINT('Ctrl Pts',(-0.217935681191677,1.67693412158597,
0.559192847558339));
#16618=CARTESIAN_POINT('Ctrl Pts',(-0.243557727551164,1.61548166177648,
0.548518231057014));
#16619=CARTESIAN_POINT('Ctrl Pts',(-0.25,1.58183602855499,0.545435605731786));
#16620=CARTESIAN_POINT('Ctrl Pts',(-0.25,1.55,0.545435605731786));
#16621=CARTESIAN_POINT('',(-0.25,1.55,0.));
#16622=CARTESIAN_POINT('Origin',(1.65,2.25,0.));
#16623=CARTESIAN_POINT('',(-0.6,2.25,-7.34788079488412E-17));
#16624=CARTESIAN_POINT('Origin',(0.,2.25,0.));
#16625=CARTESIAN_POINT('Origin',(1.75,0.85,0.));
#16626=CARTESIAN_POINT('',(-1.75,0.85,-2.14313189850787E-16));
#16627=CARTESIAN_POINT('Origin',(0.,0.85,0.));
#16628=CARTESIAN_POINT('Origin',(0.,0.,0.));
#16629=CARTESIAN_POINT('',(-1.75,-0.85,-2.14313189850787E-16));
#16630=CARTESIAN_POINT('Origin',(0.,-0.85,0.));
#16631=CARTESIAN_POINT('',(-1.75,0.,-2.14313189850787E-16));
#16632=CARTESIAN_POINT('Origin',(0.6,-0.85,0.));
#16633=CARTESIAN_POINT('',(-0.6,-0.85,-7.34788079488412E-17));
#16634=CARTESIAN_POINT('Origin',(0.,-0.85,0.));
#16635=CARTESIAN_POINT('Origin',(0.,0.7,0.));
#16636=CARTESIAN_POINT('',(-0.6,0.7,-7.34788079488412E-17));
#19303=UNCERTAINTY_MEASURE_WITH_UNIT(LENGTH_MEASURE(0.001),#19362,
'DISTANCE_ACCURACY_VALUE',
'Maximum model space distance between geometric entities at asserted c
onnectivities');
#19323=UNCERTAINTY_MEASURE_WITH_UNIT(LENGTH_MEASURE(0.001),#19362,
'DISTANCE_ACCURACY_VALUE',
'Maximum model space distance between geometric entities at asserted c
onnectivities');
#19341=(
GEOMETRIC_REPRESENTATION_CONTEXT(3)
GLOBAL_UNCERTAINTY_ASSIGNED_CONTEXT((#19303))
GLOBAL_UNIT_ASSIGNED_CONTEXT((#19362,#19364,#19365))
REPRESENTATION_CONTEXT('','3D')
);
#19361=(
GEOMETRIC_REPRESENTATION_CONTEXT(3)
GLOBAL_UNCERTAINTY_ASSIGNED_CONTEXT((#19323))
GLOBAL_UNIT_ASSIGNED_CONTEXT((#19362,#19364,#19365))
REPRESENTATION_CONTEXT('','3D')
);
#19362=(
LENGTH_UNIT()
NAMED_UNIT(*)
SI_UNIT(.CENTI.,.METRE.)
);
#19364=(
NAMED_UNIT(*)
PLANE_ANGLE_UNIT()
SI_UNIT($,.RADIAN.)
);
#19365=(
NAMED_UNIT(*)
SI_UNIT($,.STERADIAN.)
SOLID_ANGLE_UNIT()
);
#19383=SHAPE_DEFINITION_REPRESENTATION(#19420,#19505);
#19420=PRODUCT_DEFINITION_SHAPE('',$,#19543);
#19505=SHAPE_REPRESENTATION('',(#11630),#19341);
#19525=PRODUCT_DEFINITION_CONTEXT('part definition',#19638,'design');
#19543=PRODUCT_DEFINITION('Insert bearing','Insert bearing',#19580,#19525);
#19580=PRODUCT_DEFINITION_FORMATION('',$,#19657);
#19638=APPLICATION_CONTEXT(
'Core Data for Automotive Mechanical Design Process');
#19639=PRODUCT_CONTEXT('part definition',#19638,'mechanical');
#19657=PRODUCT('Insert bearing','Insert bearing','Insert bearing',(#19639));
#19740=COLOUR_RGB('Grey',0.48,0.52,0.57);
#19741=FILL_AREA_STYLE_COLOUR('',#19740);
#19742=FILL_AREA_STYLE('',(#19741));
#19743=SURFACE_STYLE_FILL_AREA(#19742);
#19744=SURFACE_SIDE_STYLE('',(#19743));
#19745=SURFACE_STYLE_USAGE(.BOTH.,#19744);
#19746=PRESENTATION_STYLE_ASSIGNMENT((#19745));
ENDSEC;
END-ISO-10303-21;
